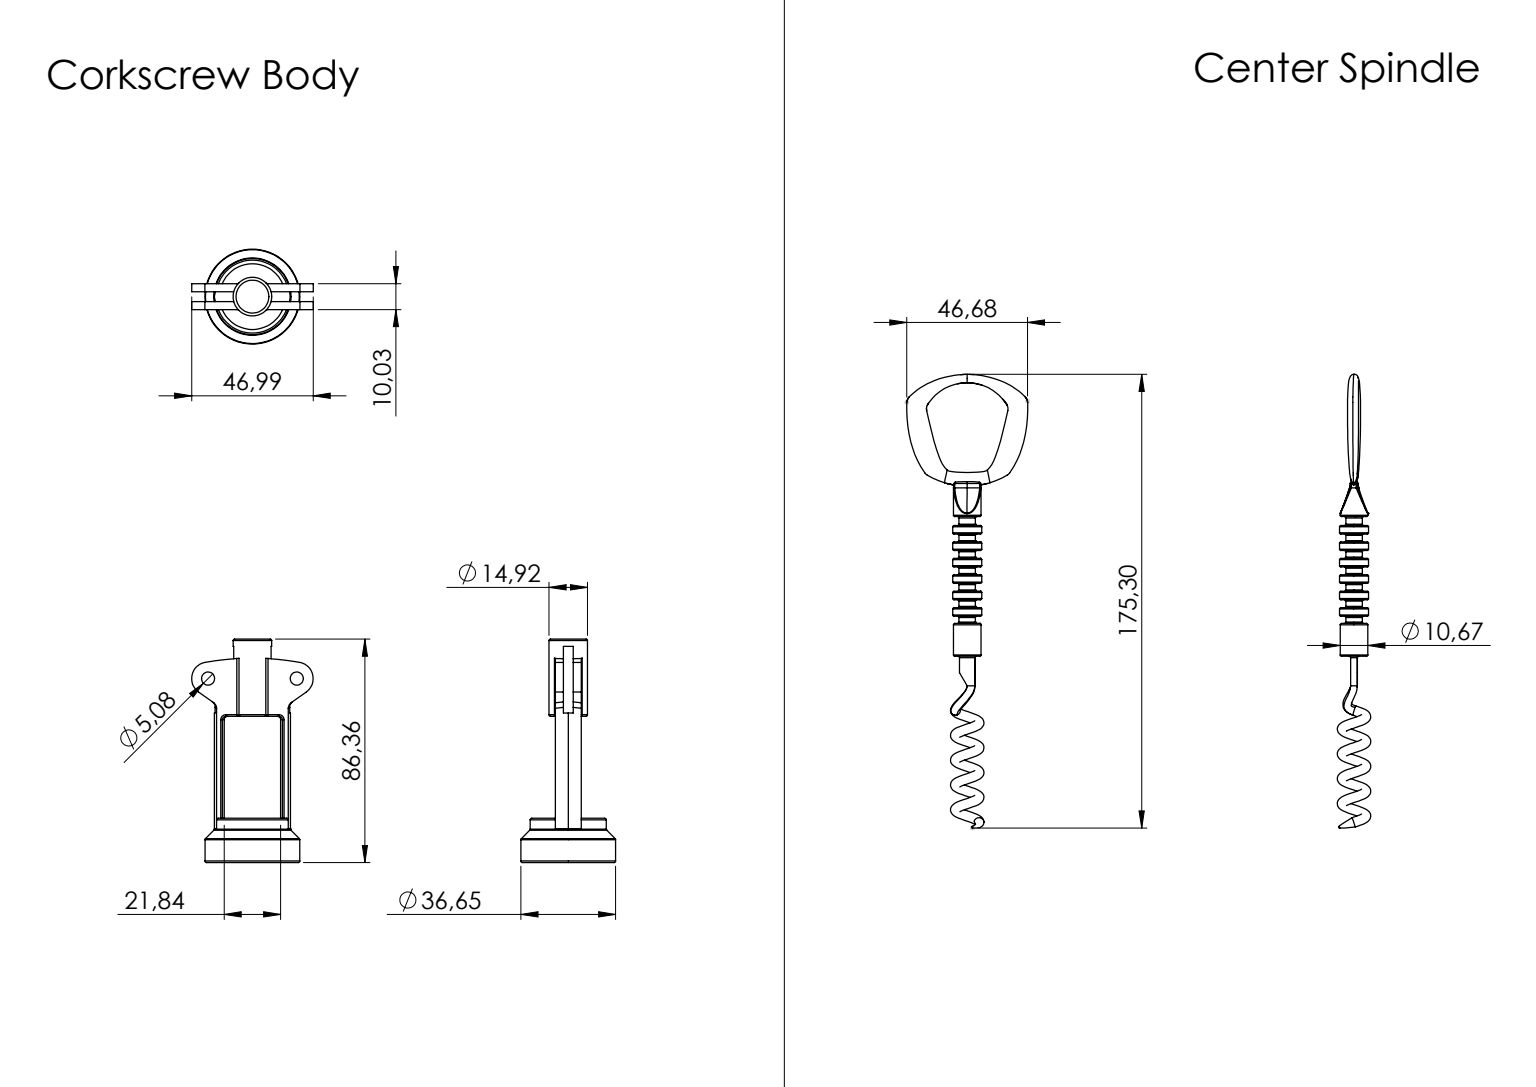
ISO-10303-21;
HEADER;
FILE_DESCRIPTION (('STEP AP214'),
    '1' );
FILE_NAME ('Corkscrew Body.step',
    '2026-10-06T14:27:08',
    ( '' ),
    ( '' ),
    'SwSTEP 2.0',
    'SolidWorks 2020',
    '' );
FILE_SCHEMA (( 'AUTOMOTIVE_DESIGN' ));
ENDSEC;

DATA;
#17=CARTESIAN_POINT ( 'NONE',  ( 16.60960244842765832, 9.026346327358513832, 0.000000000000000000 ) ) ;
#23=ORIENTED_EDGE ( 'NONE', *, *, #33925, .T. ) ;
#24=CIRCLE ( 'NONE', #38114, 2.540000000000000480 ) ;
#38=CYLINDRICAL_SURFACE ( 'NONE', #12263, 2.540000000000000480 ) ;
#46=CARTESIAN_POINT ( 'NONE',  ( -10.32169608105474090, 17.14500000000000313, 4.040823496909975887 ) ) ;
#53=DIRECTION ( 'NONE',  ( -1.000000000000000000, -9.933992704233682996E-16, 0.000000000000000000 ) ) ;
#54=CARTESIAN_POINT ( 'NONE',  ( 5.348924234570989533, 56.51499999999999346, 4.492130288940735738 ) ) ;
#63=CARTESIAN_POINT ( 'NONE',  ( 5.241362157049035631, 88.73331249999999670, 5.310945289804168468 ) ) ;
#81=AXIS2_PLACEMENT_3D ( 'NONE', #23637, #14261, #11485 ) ;
#83=CARTESIAN_POINT ( 'NONE',  ( -6.072850655491211391, 78.87349744216251679, 4.348040511725084656 ) ) ;
#86=EDGE_CURVE ( 'NONE', #35923, #21980, #18976, .T. ) ;
#92=CARTESIAN_POINT ( 'NONE',  ( 5.106395947886037234, 78.95054594174946772, -1.904999999999999583 ) ) ;
#107=VECTOR ( 'NONE', #35757, 1000.000000000000000 ) ;
#112=CARTESIAN_POINT ( 'NONE',  ( -5.241362157049125337, 53.58606250000000415, 5.310945289804168468 ) ) ;
#117=VERTEX_POINT ( 'NONE', #21192 ) ;
#125=CARTESIAN_POINT ( 'NONE',  ( 5.974493989214552769, 78.88147413144905329, -5.016499999999998849 ) ) ;
#143=CIRCLE ( 'NONE', #8295, 14.91798719394653716 ) ;
#166=ORIENTED_EDGE ( 'NONE', *, *, #11201, .F. ) ;
#183=FACE_OUTER_BOUND ( 'NONE', #18213, .T. ) ;
#195=DIRECTION ( 'NONE',  ( -1.000000000000000000, 9.627370216492861475E-17, 0.000000000000000000 ) ) ;
#199=CARTESIAN_POINT ( 'NONE',  ( -5.354045385512117505, 57.14999999999997726, -5.213862164334880589 ) ) ;
#207=PLANE ( 'NONE',  #933 ) ;
#222=CARTESIAN_POINT ( 'NONE',  ( -13.51785991797445341, 17.08228783296376818, -5.016500000000000625 ) ) ;
#244=CARTESIAN_POINT ( 'NONE',  ( -11.66725022231030628, 17.14499999999999957, -5.016499999999999737 ) ) ;
#248=ORIENTED_EDGE ( 'NONE', *, *, #30050, .T. ) ;
#268=CARTESIAN_POINT ( 'NONE',  ( -9.638062024671791406, 56.51499999999998636, 3.341163682266966022E-16 ) ) ;
#296=VERTEX_POINT ( 'NONE', #28017 ) ;
#299=ORIENTED_EDGE ( 'NONE', *, *, #22158, .F. ) ;
#305=CARTESIAN_POINT ( 'NONE',  ( -16.04309792416813707, 12.96416000000000146, 5.016499999999999737 ) ) ;
#306=ADVANCED_FACE ( 'NONE', ( #31428 ), #28233, .F. ) ;
#322=CARTESIAN_POINT ( 'NONE',  ( -5.305748947172281405, 65.30181249999996851, 5.247078976224250013 ) ) ;
#323=CARTESIAN_POINT ( 'NONE',  ( -14.73200000000000109, 57.78499999999998948, 0.000000000000000000 ) ) ;
#327=EDGE_CURVE ( 'NONE', #29906, #24559, #18939, .T. ) ;
#329=VERTEX_POINT ( 'NONE', #35268 ) ;
#344=DIRECTION ( 'NONE',  ( -1.000000000000000000, -6.353134868986659519E-16, 0.000000000000000000 ) ) ;
#359=VERTEX_POINT ( 'NONE', #29070 ) ;
#363=EDGE_CURVE ( 'NONE', #1559, #17444, #28654, .T. ) ;
#373=FACE_OUTER_BOUND ( 'NONE', #39695, .T. ) ;
#375=EDGE_CURVE ( 'NONE', #4024, #2187, #33931, .T. ) ;
#377=MECHANICAL_DESIGN_GEOMETRIC_PRESENTATION_REPRESENTATION('',(#2412),#24155);
#392=EDGE_CURVE ( 'NONE', #39604, #25560, #6092, .T. ) ;
#401=LINE ( 'NONE', #26358, #32745 ) ;
#406=EDGE_CURVE ( 'NONE', #11585, #11444, #23712, .T. ) ;
#415=CARTESIAN_POINT ( 'NONE',  ( -5.813542725971299063, 56.51499999999999346, -4.384680539058477322 ) ) ;
#431=CARTESIAN_POINT ( 'NONE',  ( -6.059261036834475256, 57.15000000000000568, 5.016499999999999737 ) ) ;
#433=EDGE_CURVE ( 'NONE', #15317, #27003, #40662, .T. ) ;
#449=VERTEX_POINT ( 'NONE', #15861 ) ;
#464=DIRECTION ( 'NONE',  ( 0.000000000000000000, 0.000000000000000000, 1.000000000000000000 ) ) ;
#479=CARTESIAN_POINT ( 'NONE',  ( -5.749535644243536581, 78.89971493812807068, 5.036102041843079746 ) ) ;
#482=CIRCLE ( 'NONE', #24259, 6.350000000000004974 ) ;
#493=ORIENTED_EDGE ( 'NONE', *, *, #10911, .T. ) ;
#506=CARTESIAN_POINT ( 'NONE',  ( -7.213960532363663525, 83.56599999999998829, -1.904999999999999805 ) ) ;
#532=CARTESIAN_POINT ( 'NONE',  ( -5.177913976931302287, 77.01756250000002524, 5.372099999999996989 ) ) ;
#552=CARTESIAN_POINT ( 'NONE',  ( 6.059261036834406866, 57.14999999999999858, -5.016499999999999737 ) ) ;
#583=CARTESIAN_POINT ( 'NONE',  ( 5.965356522962858676, 57.14999999999998437, 5.016499999999999737 ) ) ;
#584=ORIENTED_EDGE ( 'NONE', *, *, #327, .T. ) ;
#585=FACE_BOUND ( 'NONE', #36365, .T. ) ;
#586=EDGE_CURVE ( 'NONE', #26988, #6334, #37150, .T. ) ;
#605=CARTESIAN_POINT ( 'NONE',  ( 6.059261036834405978, 57.14999999999999858, 5.016500000000000625 ) ) ;
#609=CARTESIAN_POINT ( 'NONE',  ( -5.177913976931298734, 78.94499979771843812, 5.372100000000002318 ) ) ;
#619=ORIENTED_EDGE ( 'NONE', *, *, #5064, .T. ) ;
#627=CARTESIAN_POINT ( 'NONE',  ( -6.059261036834475256, 57.14999999999997016, -5.016499999999997961 ) ) ;
#644=EDGE_CURVE ( 'NONE', #33497, #18509, #30539, .T. ) ;
#660=ORIENTED_EDGE ( 'NONE', *, *, #1717, .T. ) ;
#672=ORIENTED_EDGE ( 'NONE', *, *, #20953, .T. ) ;
#676=DIRECTION ( 'NONE',  ( 6.353134868986659519E-16, -1.000000000000000000, -0.000000000000000000 ) ) ;
#677=EDGE_CURVE ( 'NONE', #32690, #22720, #25591, .T. ) ;
#681=CARTESIAN_POINT ( 'NONE',  ( 11.42297701379736097, 55.88459609804032624, 4.463034230327253660 ) ) ;
#688=CARTESIAN_POINT ( 'NONE',  ( -6.057513928997661168, 86.35999999999998522, 1.904999999999996030 ) ) ;
#700=VERTEX_POINT ( 'NONE', #35196 ) ;
#737=VECTOR ( 'NONE', #34279, 1000.000000000000000 ) ;
#738=EDGE_CURVE ( 'NONE', #20977, #19747, #15581, .T. ) ;
#739=CARTESIAN_POINT ( 'NONE',  ( -5.706177858098648414, 57.14999999999999147, 5.041924732081957572 ) ) ;
#740=CARTESIAN_POINT ( 'NONE',  ( -14.50851225146815615, 78.09971119798315442, -5.392902600000144986 ) ) ;
#747=ORIENTED_EDGE ( 'NONE', *, *, #36377, .F. ) ;
#772=ORIENTED_EDGE ( 'NONE', *, *, #41947, .T. ) ;
#798=CARTESIAN_POINT ( 'NONE',  ( 10.92199999999999704, 56.51500000000000057, 5.016499999999999737 ) ) ;
#815=EDGE_LOOP ( 'NONE', ( #35010, #24388, #10696, #2697 ) ) ;
#829=CARTESIAN_POINT ( 'NONE',  ( -18.10310074716289819, 60.88085900918027704, 4.514343177587270439 ) ) ;
#830=EDGE_CURVE ( 'NONE', #3380, #4530, #15208, .T. ) ;
#841=ORIENTED_EDGE ( 'NONE', *, *, #41067, .T. ) ;
#859=CARTESIAN_POINT ( 'NONE',  ( 5.965356522962838248, 88.73331249999999670, -5.016499999999999737 ) ) ;
#877=EDGE_CURVE ( 'NONE', #14016, #35273, #12805, .T. ) ;
#879=VECTOR ( 'NONE', #18768, 1000.000000000000000 ) ;
#883=CARTESIAN_POINT ( 'NONE',  ( 5.177913976931214357, 57.15000000000004832, 5.372099999999999653 ) ) ;
#884=ADVANCED_FACE ( 'NONE', ( #39437, #36878 ), #33047, .F. ) ;
#896=CARTESIAN_POINT ( 'NONE',  ( -5.285751105923923276, 78.93631598568865115, 5.267410652559463280 ) ) ;
#899=AXIS2_PLACEMENT_3D ( 'NONE', #27632, #8047, #4662 ) ;
#906=AXIS2_PLACEMENT_3D ( 'NONE', #17827, #7426, #24216 ) ;
#914=EDGE_CURVE ( 'NONE', #2471, #24940, #10804, .T. ) ;
#920=ADVANCED_FACE ( 'NONE', ( #1310 ), #35822, .T. ) ;
#922=AXIS2_PLACEMENT_3D ( 'NONE', #6804, #22543, #10198 ) ;
#926=VERTEX_POINT ( 'NONE', #17468 ) ;
#931=EDGE_CURVE ( 'NONE', #32109, #25746, #26433, .T. ) ;
#932=CARTESIAN_POINT ( 'NONE',  ( 11.11710224467026542, 56.30409367656755393, -5.016499999999892268 ) ) ;
#933=AXIS2_PLACEMENT_3D ( 'NONE', #16577, #26595, #39603 ) ;
#934=ADVANCED_FACE ( 'NONE', ( #10661 ), #17435, .T. ) ;
#950=CARTESIAN_POINT ( 'NONE',  ( -4.965996940879724875, 56.51500000000000767, 4.710730864944216556 ) ) ;
#970=DIRECTION ( 'NONE',  ( -0.8138664877804109299, 0.5810519254489895369, 0.000000000000000000 ) ) ;
#1007=VERTEX_POINT ( 'NONE', #36453 ) ;
#1017=CARTESIAN_POINT ( 'NONE',  ( 6.059261036833978764, 78.87450423423040036, 5.016499999999999737 ) ) ;
#1029=ORIENTED_EDGE ( 'NONE', *, *, #32030, .T. ) ;
#1042=COLOUR_RGB ( '', 0.08235294, 0.09019608, 0.10196078) ;
#1052=ORIENTED_EDGE ( 'NONE', *, *, #4297, .T. ) ;
#1067=CARTESIAN_POINT ( 'NONE',  ( 5.475330206976798841, 65.30181249999998272, -5.107412922131463695 ) ) ;
#1086=EDGE_CURVE ( 'NONE', #24253, #32761, #16627, .T. ) ;
#1089=CYLINDRICAL_SURFACE ( 'NONE', #27471, 14.73199999999999577 ) ;
#1109=CARTESIAN_POINT ( 'NONE',  ( -5.153324091253895567, 56.51694919289731445, -4.640537933314518249 ) ) ;
#1121=EDGE_LOOP ( 'NONE', ( #34298, #24074 ) ) ;
#1132=ADVANCED_FACE ( 'NONE', ( #40076 ), #32397, .T. ) ;
#1152=FACE_OUTER_BOUND ( 'NONE', #15557, .T. ) ;
#1157=LINE ( 'NONE', #36934, #4914 ) ;
#1161=VECTOR ( 'NONE', #11393, 1000.000000000000000 ) ;
#1166=ORIENTED_EDGE ( 'NONE', *, *, #32177, .F. ) ;
#1177=CARTESIAN_POINT ( 'NONE',  ( -14.73199999999999754, 61.59499999999999886, 5.016499999999999737 ) ) ;
#1205=EDGE_CURVE ( 'NONE', #21382, #34762, #21073, .T. ) ;
#1209=CARTESIAN_POINT ( 'NONE',  ( -11.66725022231030984, 16.50999999999999801, 5.016499999999999737 ) ) ;
#1242=ORIENTED_EDGE ( 'NONE', *, *, #38846, .T. ) ;
#1250=CARTESIAN_POINT ( 'NONE',  ( 14.60500000000000043, 71.11999999999999034, -1.904999999999999583 ) ) ;
#1264=FACE_OUTER_BOUND ( 'NONE', #33978, .T. ) ;
#1296=DIRECTION ( 'NONE',  ( 9.627370216492862708E-17, 1.000000000000000000, -0.000000000000000000 ) ) ;
#1307=CYLINDRICAL_SURFACE ( 'NONE', #5741, 18.32410244842765934 ) ;
#1308=VECTOR ( 'NONE', #32914, 1000.000000000000000 ) ;
#1310=FACE_OUTER_BOUND ( 'NONE', #18095, .T. ) ;
#1313=ORIENTED_EDGE ( 'NONE', *, *, #40737, .T. ) ;
#1327=ORIENTED_EDGE ( 'NONE', *, *, #33725, .F. ) ;
#1357=AXIS2_PLACEMENT_3D ( 'NONE', #16330, #30595, #17389 ) ;
#1371=ORIENTED_EDGE ( 'NONE', *, *, #327, .F. ) ;
#1374=VERTEX_POINT ( 'NONE', #11919 ) ;
#1386=ORIENTED_EDGE ( 'NONE', *, *, #433, .F. ) ;
#1397=VERTEX_POINT ( 'NONE', #25016 ) ;
#1404=DIRECTION ( 'NONE',  ( -0.000000000000000000, -0.000000000000000000, -1.000000000000000000 ) ) ;
#1422=VERTEX_POINT ( 'NONE', #19455 ) ;
#1427=PLANE ( 'NONE',  #33605 ) ;
#1454=FACE_OUTER_BOUND ( 'NONE', #20510, .T. ) ;
#1460=DIRECTION ( 'NONE',  ( -1.000000000000000000, 0.000000000000000000, 0.000000000000000000 ) ) ;
#1463=EDGE_CURVE ( 'NONE', #18019, #32240, #9670, .T. ) ;
#1466=AXIS2_PLACEMENT_3D ( 'NONE', #18039, #21025, #19252 ) ;
#1485=DIRECTION ( 'NONE',  ( 9.627370216492862708E-17, 1.000000000000000000, -0.000000000000000000 ) ) ;
#1489=CARTESIAN_POINT ( 'NONE',  ( 5.965356522962860453, 65.30181249999998272, -5.016499999999999737 ) ) ;
#1511=ORIENTED_EDGE ( 'NONE', *, *, #11811, .F. ) ;
#1514=CARTESIAN_POINT ( 'NONE',  ( 12.21488373879589240, 17.14499999999999957, 4.381499999999999950 ) ) ;
#1519=CARTESIAN_POINT ( 'NONE',  ( 9.925711944554073796, 78.55658865046544292, -5.016499999999999737 ) ) ;
#1529=CARTESIAN_POINT ( 'NONE',  ( -11.37822013471355653, 56.06794068206369275, -5.016499999999995296 ) ) ;
#1531=CIRCLE ( 'NONE', #25317, 18.13811525448111439 ) ;
#1533=CARTESIAN_POINT ( 'NONE',  ( 1.247998466936322838E-15, 12.96302561210691806, 0.000000000000000000 ) ) ;
#1544=VERTEX_POINT ( 'NONE', #29261 ) ;
#1559=VERTEX_POINT ( 'NONE', #16682 ) ;
#1561=CARTESIAN_POINT ( 'NONE',  ( 10.45722248778832508, 56.52709681235301531, -5.016500000000866599 ) ) ;
#1573=VECTOR ( 'NONE', #21848, 999.9999999999998863 ) ;
#1616=DIRECTION ( 'NONE',  ( -1.000000000000000000, -6.353134868986659519E-16, 6.146657985744592735E-16 ) ) ;
#1628=ORIENTED_EDGE ( 'NONE', *, *, #19844, .T. ) ;
#1638=LINE ( 'NONE', #34216, #5021 ) ;
#1675=AXIS2_PLACEMENT_3D ( 'NONE', #6302, #35478, #19903 ) ;
#1699=DIRECTION ( 'NONE',  ( 0.1469470846586743706, 0.000000000000000000, 0.9891443546370348727 ) ) ;
#1717=EDGE_CURVE ( 'NONE', #31005, #40327, #26908, .T. ) ;
#1727=ADVANCED_FACE ( 'NONE', ( #1152 ), #40132, .T. ) ;
#1735=DIRECTION ( 'NONE',  ( -1.000000000000000000, 0.000000000000000000, -6.146657985744586818E-16 ) ) ;
#1749=EDGE_CURVE ( 'NONE', #19747, #35348, #13067, .T. ) ;
#1755=FILL_AREA_STYLE_COLOUR ( '', #18907 ) ;
#1769=AXIS2_PLACEMENT_3D ( 'NONE', #10155, #36381, #23767 ) ;
#1787=CARTESIAN_POINT ( 'NONE',  ( 4.792324638223571576, 56.51998046905274009, -4.972049999999996750 ) ) ;
#1816=LINE ( 'NONE', #30764, #8889 ) ;
#1830=ORIENTED_EDGE ( 'NONE', *, *, #17540, .F. ) ;
#1833=DIRECTION ( 'NONE',  ( -0.000000000000000000, -0.000000000000000000, -1.000000000000000000 ) ) ;
#1848=DIRECTION ( 'NONE',  ( -1.000000000000000000, -5.463695987328526437E-16, 0.000000000000000000 ) ) ;
#1874=DIRECTION ( 'NONE',  ( -0.000000000000000000, -0.000000000000000000, -1.000000000000000000 ) ) ;
#1876=CARTESIAN_POINT ( 'NONE',  ( 6.059261036834405978, 56.51500000000000057, -5.016500000000000625 ) ) ;
#1883=VERTEX_POINT ( 'NONE', #18570 ) ;
#1892=ORIENTED_EDGE ( 'NONE', *, *, #31827, .F. ) ;
#1907=VECTOR ( 'NONE', #2855, 1000.000000000000000 ) ;
#1910=ADVANCED_FACE ( 'NONE', ( #37755 ), #18355, .F. ) ;
#1923=DIRECTION ( 'NONE',  ( -1.000000000000000000, 0.000000000000000000, 0.000000000000000000 ) ) ;
#1930=CARTESIAN_POINT ( 'NONE',  ( -5.177913976931281859, 56.51500000000002899, -5.372099999999998765 ) ) ;
#1935=CYLINDRICAL_SURFACE ( 'NONE', #12373, 2.539999999999999591 ) ;
#1942=CARTESIAN_POINT ( 'NONE',  ( -11.66725022231030628, 55.24499999999998323, -5.016500000000000625 ) ) ;
#1962=SURFACE_SIDE_STYLE ('',( #8555 ) ) ;
#1964=DIRECTION ( 'NONE',  ( 1.000000000000000000, 0.000000000000000000, 1.224646799147353207E-16 ) ) ;
#1968=DIRECTION ( 'NONE',  ( -6.353134868986659519E-16, 1.000000000000000000, 0.000000000000000000 ) ) ;
#1976=FACE_OUTER_BOUND ( 'NONE', #17302, .T. ) ;
#2000=CIRCLE ( 'NONE', #24436, 12.69999999999999751 ) ;
#2012=DIRECTION ( 'NONE',  ( 0.9849462604886048966, -0.000000000000000000, 0.1728608224830406881 ) ) ;
#2044=ORIENTED_EDGE ( 'NONE', *, *, #9457, .T. ) ;
#2049=CARTESIAN_POINT ( 'NONE',  ( 5.230039278750658660, 78.94094791484917550, -5.321858878493932465 ) ) ;
#2057=CARTESIAN_POINT ( 'NONE',  ( -5.817775060672866871, 56.51499999999999346, -4.384522920466269014 ) ) ;
#2074=ORIENTED_EDGE ( 'NONE', *, *, #375, .F. ) ;
#2078=FACE_OUTER_BOUND ( 'NONE', #34790, .T. ) ;
#2083=EDGE_CURVE ( 'NONE', #14687, #5970, #12181, .T. ) ;
#2085=CARTESIAN_POINT ( 'NONE',  ( 5.115576404397946142, 56.51499999999996504, -4.603576161448420301 ) ) ;
#2088=VECTOR ( 'NONE', #7580, 1000.000000000000227 ) ;
#2098=DIRECTION ( 'NONE',  ( -1.000000000000000000, 0.000000000000000000, 0.000000000000000000 ) ) ;
#2108=DIRECTION ( 'NONE',  ( 0.8138664877804110409, 0.5810519254489896479, -5.002558946445370251E-16 ) ) ;
#2110=LINE ( 'NONE', #34903, #737 ) ;
#2132=FACE_OUTER_BOUND ( 'NONE', #16740, .T. ) ;
#2134=EDGE_CURVE ( 'NONE', #25560, #18746, #14952, .T. ) ;
#2138=CIRCLE ( 'NONE', #30043, 12.69999999999999751 ) ;
#2141=CARTESIAN_POINT ( 'NONE',  ( -14.73199999999999399, 12.96302561210691984, 0.000000000000000000 ) ) ;
#2145=ORIENTED_EDGE ( 'NONE', *, *, #40646, .F. ) ;
#2146=DIRECTION ( 'NONE',  ( -1.000000000000000000, 0.000000000000000000, 0.000000000000000000 ) ) ;
#2150=DIRECTION ( 'NONE',  ( 0.000000000000000000, 0.000000000000000000, -1.000000000000000000 ) ) ;
#2153=LINE ( 'NONE', #15113, #21689 ) ;
#2164=EDGE_LOOP ( 'NONE', ( #13314, #38087, #29660, #7685 ) ) ;
#2177=DIRECTION ( 'NONE',  ( -0.9849462604886047856, 0.000000000000000000, -0.1728608224830407714 ) ) ;
#2187=VERTEX_POINT ( 'NONE', #12611 ) ;
#2189=FACE_OUTER_BOUND ( 'NONE', #17505, .T. ) ;
#2204=DIRECTION ( 'NONE',  ( -1.000000000000000000, 0.000000000000000000, 0.000000000000000000 ) ) ;
#2209=CARTESIAN_POINT ( 'NONE',  ( 5.177913976931212581, 57.15000000000004832, -5.372100000000001430 ) ) ;
#2215=AXIS2_PLACEMENT_3D ( 'NONE', #11347, #15162, #11767 ) ;
#2216=ORIENTED_EDGE ( 'NONE', *, *, #20706, .T. ) ;
#2248=CARTESIAN_POINT ( 'NONE',  ( -6.985000000000036735, 57.14999999999998437, 0.000000000000000000 ) ) ;
#2252=LINE ( 'NONE', #11602, #31088 ) ;
#2260=FACE_OUTER_BOUND ( 'NONE', #37704, .T. ) ;
#2266=DIRECTION ( 'NONE',  ( 1.000000000000000000, -1.162840169671635117E-16, 0.000000000000000000 ) ) ;
#2274=CARTESIAN_POINT ( 'NONE',  ( 5.177913976931196594, 78.94499979771845233, -5.372100000000001430 ) ) ;
#2296=VECTOR ( 'NONE', #9251, 1000.000000000000000 ) ;
#2302=CARTESIAN_POINT ( 'NONE',  ( 5.860205464978446521, 56.51500000000089585, -5.019550312247728741 ) ) ;
#2314=CARTESIAN_POINT ( 'NONE',  ( -17.68910244842765778, 8.844871939465427602, 2.166290269325653984E-15 ) ) ;
#2341=VECTOR ( 'NONE', #1296, 1000.000000000000000 ) ;
#2349=AXIS2_PLACEMENT_3D ( 'NONE', #22246, #26089, #344 ) ;
#2350=PLANE ( 'NONE',  #8239 ) ;
#2354=CARTESIAN_POINT ( 'NONE',  ( -12.16475753114683656, 55.74362973025081658, 5.016499999999999737 ) ) ;
#2357=DIRECTION ( 'NONE',  ( -1.000000000000000000, -9.933992704233682996E-16, 0.000000000000000000 ) ) ;
#2359=ORIENTED_EDGE ( 'NONE', *, *, #37833, .F. ) ;
#2369=DIRECTION ( 'NONE',  ( -1.224646799147353207E-16, 1.179012811983454535E-32, 1.000000000000000000 ) ) ;
#2378=ORIENTED_EDGE ( 'NONE', *, *, #677, .T. ) ;
#2384=EDGE_CURVE ( 'NONE', #36071, #117, #19612, .T. ) ;
#2391=DIRECTION ( 'NONE',  ( 6.353134868986659519E-16, -1.000000000000000000, 0.000000000000000000 ) ) ;
#2411=EDGE_CURVE ( 'NONE', #7919, #11738, #39022, .T. ) ;
#2412=STYLED_ITEM ( 'NONE', ( #26181 ), #38952 ) ;
#2421=CARTESIAN_POINT ( 'NONE',  ( 10.92199999999999704, 16.51000000000000156, 5.016499999999999737 ) ) ;
#2425=ORIENTED_EDGE ( 'NONE', *, *, #35443, .F. ) ;
#2440=B_SPLINE_SURFACE_WITH_KNOTS ( 'NONE', 3, 1, ( 
 ( #6364, #2966 ),
 ( #22726, #38531 ),
 ( #26158, #13168 ),
 ( #15929, #28725 ) ),
 .UNSPECIFIED., .F., .F., .F.,
 ( 4, 4 ),
 ( 2, 2 ),
 ( 0.000000000000000000, 0.6118630412642164229 ),
 ( 0.000000000000000000, 1.000000000000000000 ),
 .UNSPECIFIED. ) ;
#2448=ORIENTED_EDGE ( 'NONE', *, *, #21122, .T. ) ;
#2466=EDGE_CURVE ( 'NONE', #35912, #359, #33547, .T. ) ;
#2467=CARTESIAN_POINT ( 'NONE',  ( -5.965356522962950159, 77.01756249999996840, -5.016499999999999737 ) ) ;
#2470=VECTOR ( 'NONE', #25773, 999.9999999999998863 ) ;
#2471=VERTEX_POINT ( 'NONE', #33268 ) ;
#2474=DIRECTION ( 'NONE',  ( -1.000000000000000000, 9.627370216492862708E-17, 0.000000000000000000 ) ) ;
#2480=DIRECTION ( 'NONE',  ( 0.000000000000000000, 0.000000000000000000, -1.000000000000000000 ) ) ;
#2487=PLANE ( 'NONE',  #4772 ) ;
#2488=EDGE_CURVE ( 'NONE', #18952, #41795, #38005, .T. ) ;
#2517=CARTESIAN_POINT ( 'NONE',  ( 5.652760403059779115, 78.90762248850970195, 4.881857480398483773 ) ) ;
#2518=EDGE_CURVE ( 'NONE', #38485, #22696, #17475, .T. ) ;
#2521=EDGE_CURVE ( 'NONE', #19034, #29525, #10668, .T. ) ;
#2547=ORIENTED_EDGE ( 'NONE', *, *, #22871, .F. ) ;
#2554=VECTOR ( 'NONE', #26088, 1000.000000000000000 ) ;
#2559=CARTESIAN_POINT ( 'NONE',  ( 1.650612623617701454E-15, 17.14499999999999957, 0.000000000000000000 ) ) ;
#2560=AXIS2_PLACEMENT_3D ( 'NONE', #26322, #10762, #36974 ) ;
#2561=DIRECTION ( 'NONE',  ( 0.000000000000000000, -0.000000000000000000, -1.000000000000000000 ) ) ;
#2567=CARTESIAN_POINT ( 'NONE',  ( 5.237865101059586692, 78.94033958618257429, 5.314315937239232568 ) ) ;
#2583=DIRECTION ( 'NONE',  ( -0.000000000000000000, -0.000000000000000000, -1.000000000000000000 ) ) ;
#2628=CARTESIAN_POINT ( 'NONE',  ( -5.266289895157169814E-14, 83.56599999999998829, 1.904999999999999805 ) ) ;
#2631=PLANE ( 'NONE',  #39625 ) ;
#2695=CARTESIAN_POINT ( 'NONE',  ( 12.21488373879589240, 71.11999999999999034, 5.016499999999999737 ) ) ;
#2696=CARTESIAN_POINT ( 'NONE',  ( 5.177913976931201923, 71.67999986514567468, -5.372100000000002318 ) ) ;
#2697=ORIENTED_EDGE ( 'NONE', *, *, #29178, .F. ) ;
#2707=EDGE_CURVE ( 'NONE', #32109, #11189, #16941, .T. ) ;
#2711=AXIS2_PLACEMENT_3D ( 'NONE', #25509, #5513, #21659 ) ;
#2719=DIRECTION ( 'NONE',  ( -0.000000000000000000, -0.000000000000000000, -1.000000000000000000 ) ) ;
#2724=CARTESIAN_POINT ( 'NONE',  ( 5.353961913965608055, 57.14999999999869829, -5.213928161019547147 ) ) ;
#2728=FACE_OUTER_BOUND ( 'NONE', #31465, .T. ) ;
#2731=CIRCLE ( 'NONE', #26532, 12.69999999999999751 ) ;
#2754=ORIENTED_EDGE ( 'NONE', *, *, #4976, .F. ) ;
#2757=EDGE_CURVE ( 'NONE', #3380, #22739, #11186, .T. ) ;
#2767=ADVANCED_FACE ( 'NONE', ( #33780 ), #30564, .F. ) ;
#2771=CARTESIAN_POINT ( 'NONE',  ( -11.58677707360117282, 55.41127257906216386, 4.474811398756911807 ) ) ;
#2772=CARTESIAN_POINT ( 'NONE',  ( 5.624629865489175096, 78.90958242041968163, 5.067363953418781541 ) ) ;
#2776=CARTESIAN_POINT ( 'NONE',  ( 18.10310074716289819, 60.88085900918027704, 4.514343177587270439 ) ) ;
#2779=ORIENTED_EDGE ( 'NONE', *, *, #9655, .T. ) ;
#2792=FILL_AREA_STYLE_COLOUR ( '', #1042 ) ;
#2794=CARTESIAN_POINT ( 'NONE',  ( -6.985000000000036735, 56.51499999999998636, 0.000000000000000000 ) ) ;
#2803=ORIENTED_EDGE ( 'NONE', *, *, #2521, .F. ) ;
#2804=EDGE_LOOP ( 'NONE', ( #15092, #6381, #25239, #7806 ) ) ;
#2819=AXIS2_PLACEMENT_3D ( 'NONE', #38175, #21956, #5807 ) ;
#2827=CARTESIAN_POINT ( 'NONE',  ( -5.177913976931298734, 78.94499979771843812, -5.372100000000003206 ) ) ;
#2834=CARTESIAN_POINT ( 'NONE',  ( -10.39017547737320157, 56.51499999999998636, 6.098637220230963427E-16 ) ) ;
#2838=DIRECTION ( 'NONE',  ( 1.000000000000000000, 0.000000000000000000, 0.000000000000000000 ) ) ;
#2852=ORIENTED_EDGE ( 'NONE', *, *, #6404, .T. ) ;
#2855=DIRECTION ( 'NONE',  ( 0.000000000000000000, 1.000000000000000000, 0.000000000000000000 ) ) ;
#2857=CARTESIAN_POINT ( 'NONE',  ( 17.14499999999999957, 71.11999999999999034, 5.016499999999999737 ) ) ;
#2862=ORIENTED_EDGE ( 'NONE', *, *, #3971, .T. ) ;
#2869=CARTESIAN_POINT ( 'NONE',  ( 14.50851225146812240, 78.09971119798316863, -1.904999999999999583 ) ) ;
#2872=DIRECTION ( 'NONE',  ( 6.353134868986659519E-16, -1.000000000000000000, 0.000000000000000000 ) ) ;
#2882=CARTESIAN_POINT ( 'NONE',  ( -5.475330206976867231, 65.30181249999998272, -5.107412922131463695 ) ) ;
#2888=EDGE_CURVE ( 'NONE', #8736, #12419, #14571, .T. ) ;
#2895=DIRECTION ( 'NONE',  ( -9.627370216492862708E-17, -1.000000000000000000, 0.000000000000000000 ) ) ;
#2899=CARTESIAN_POINT ( 'NONE',  ( 10.86251533436410277, 78.45482716897161879, 1.904999999999999583 ) ) ;
#2905=EDGE_LOOP ( 'NONE', ( #38246, #11736, #28782, #1830 ) ) ;
#2912=EDGE_CURVE ( 'NONE', #2187, #21980, #1816, .T. ) ;
#2918=CARTESIAN_POINT ( 'NONE',  ( -10.92199999999999704, 12.96416000000000146, 0.000000000000000000 ) ) ;
#2920=ORIENTED_EDGE ( 'NONE', *, *, #2488, .F. ) ;
#2934=ORIENTED_EDGE ( 'NONE', *, *, #1749, .T. ) ;
#2952=AXIS2_PLACEMENT_3D ( 'NONE', #5972, #19351, #38343 ) ;
#2966=CARTESIAN_POINT ( 'NONE',  ( 18.35410564743290962, 77.35382415001784295, 1.904999999999988258 ) ) ;
#2972=CARTESIAN_POINT ( 'NONE',  ( -5.449227423685445437, 56.51500000000039847, -5.145694933558188744 ) ) ;
#2975=CARTESIAN_POINT ( 'NONE',  ( 5.654802103384407808, 78.90710107780496685, 5.057831774704117045 ) ) ;
#2997=CARTESIAN_POINT ( 'NONE',  ( -9.665786669610962889, 55.24499999999999034, 0.1866227975165204167 ) ) ;
#3003=DIRECTION ( 'NONE',  ( -1.000000000000000000, 1.288607544181256696E-16, 0.000000000000000000 ) ) ;
#3029=EDGE_CURVE ( 'NONE', #14963, #32351, #15483, .T. ) ;
#3030=DIRECTION ( 'NONE',  ( -1.000000000000000000, 0.000000000000000000, 0.000000000000000000 ) ) ;
#3036=CARTESIAN_POINT ( 'NONE',  ( -11.58677707360137532, 17.14499999999999957, 4.474811398758258285 ) ) ;
#3052=ORIENTED_EDGE ( 'NONE', *, *, #1205, .T. ) ;
#3054=( BOUNDED_CURVE ( )  B_SPLINE_CURVE ( 3, ( #28704, #41713, #12519, #28909 ),
 .UNSPECIFIED., .F., .T. ) 
 B_SPLINE_CURVE_WITH_KNOTS ( ( 4, 4 ),
 ( 4.712388980384686121, 5.673871460451326065 ),
 .UNSPECIFIED. ) 
 CURVE ( )  GEOMETRIC_REPRESENTATION_ITEM ( )  RATIONAL_B_SPLINE_CURVE ( ( 1.000000000000000000, 0.9244349266169030743, 0.9244349266169030743, 1.000000000000000000 ) ) 
 REPRESENTATION_ITEM ( '' )  );
#3062=ORIENTED_EDGE ( 'NONE', *, *, #26982, .T. ) ;
#3074=ORIENTED_EDGE ( 'NONE', *, *, #3776, .T. ) ;
#3090=LINE ( 'NONE', #19457, #7963 ) ;
#3110=CARTESIAN_POINT ( 'NONE',  ( -10.92199999999999704, 55.24499999999999034, -7.690731210240437325E-16 ) ) ;
#3156=CARTESIAN_POINT ( 'NONE',  ( 4.825844303143274949, 56.51499999999997215, 4.829557277217847222 ) ) ;
#3161=ORIENTED_EDGE ( 'NONE', *, *, #5173, .T. ) ;
#3167=VERTEX_POINT ( 'NONE', #323 ) ;
#3169=DIRECTION ( 'NONE',  ( -1.000000000000000000, -6.353134868986659519E-16, 0.000000000000000000 ) ) ;
#3176=CARTESIAN_POINT ( 'NONE',  ( 5.594725610051233922, 78.91206791035247647, 5.077866005995121057 ) ) ;
#3183=FACE_BOUND ( 'NONE', #18284, .T. ) ;
#3184=AXIS2_PLACEMENT_3D ( 'NONE', #23963, #20974, #13964 ) ;
#3185=ORIENTED_EDGE ( 'NONE', *, *, #35246, .F. ) ;
#3193=CARTESIAN_POINT ( 'NONE',  ( -6.059261036834476144, 56.58343591620776181, 4.712961528314683513 ) ) ;
#3198=FACE_OUTER_BOUND ( 'NONE', #31075, .T. ) ;
#3225=ADVANCED_FACE ( 'NONE', ( #2728 ), #13858, .T. ) ;
#3228=ORIENTED_EDGE ( 'NONE', *, *, #6639, .F. ) ;
#3231=LINE ( 'NONE', #13229, #9569 ) ;
#3234=CARTESIAN_POINT ( 'NONE',  ( -16.04309792416813707, 12.96416000000000146, 5.016499999999999737 ) ) ;
#3239=DIRECTION ( 'NONE',  ( 0.1469470846586743706, -1.414713986243376972E-17, 0.9891443546370348727 ) ) ;
#3251=DIRECTION ( 'NONE',  ( 9.627370216492862708E-17, 1.000000000000000000, -0.000000000000000000 ) ) ;
#3255=CIRCLE ( 'NONE', #27716, 6.350000000000004974 ) ;
#3259=DIRECTION ( 'NONE',  ( 6.353134868986659519E-16, -1.000000000000000000, 0.000000000000000000 ) ) ;
#3269=DIRECTION ( 'NONE',  ( -1.000000000000000000, 1.044409991968846932E-16, 0.000000000000000000 ) ) ;
#3274=CARTESIAN_POINT ( 'NONE',  ( -5.653927021192587610, 78.90752773945908416, 4.880377097574616130 ) ) ;
#3275=AXIS2_PLACEMENT_3D ( 'NONE', #6670, #19223, #39468 ) ;
#3284=CARTESIAN_POINT ( 'NONE',  ( 14.50851225146812240, 78.09971119798316863, -5.392902600000141433 ) ) ;
#3292=ORIENTED_EDGE ( 'NONE', *, *, #3466, .T. ) ;
#3321=DIRECTION ( 'NONE',  ( -0.1469470846586743706, 1.414713986243376972E-17, -0.9891443546370348727 ) ) ;
#3326=AXIS2_PLACEMENT_3D ( 'NONE', #13453, #16635, #4514 ) ;
#3339=ORIENTED_EDGE ( 'NONE', *, *, #25682, .F. ) ;
#3363=LINE ( 'NONE', #6762, #28527 ) ;
#3365=AXIS2_PLACEMENT_3D ( 'NONE', #37717, #35158, #38560 ) ;
#3370=CARTESIAN_POINT ( 'NONE',  ( 5.449227423779250401, 57.14999999999996305, 5.145694933688582218 ) ) ;
#3377=DIRECTION ( 'NONE',  ( 1.000000000000000000, 1.004817652842027660E-15, 0.000000000000000000 ) ) ;
#3379=ADVANCED_FACE ( 'NONE', ( #14538 ), #7331, .F. ) ;
#3380=VERTEX_POINT ( 'NONE', #37341 ) ;
#3382=CARTESIAN_POINT ( 'NONE',  ( 6.113380087472956159E-17, 0.6350000000000001199, 0.000000000000000000 ) ) ;
#3388=CARTESIAN_POINT ( 'NONE',  ( -13.85159022459153988, 59.63164443796365077, 5.016499999999999737 ) ) ;
#3391=CARTESIAN_POINT ( 'NONE',  ( 5.736468567008338404, 78.90050738914777639, 5.037638016205330693 ) ) ;
#3392=CARTESIAN_POINT ( 'NONE',  ( 16.04309792416813707, 12.96416000000000146, 5.016499999999999737 ) ) ;
#3396=CARTESIAN_POINT ( 'NONE',  ( -5.654802103384504619, 78.90710107780492422, -5.057831774704119709 ) ) ;
#3409=CARTESIAN_POINT ( 'NONE',  ( -13.83234216238653858, 16.68269501491596785, -5.016499999999998849 ) ) ;
#3424=EDGE_CURVE ( 'NONE', #33118, #4862, #30711, .T. ) ;
#3426=ORIENTED_EDGE ( 'NONE', *, *, #30280, .F. ) ;
#3434=EDGE_CURVE ( 'NONE', #31942, #3896, #27315, .T. ) ;
#3445=CYLINDRICAL_SURFACE ( 'NONE', #40339, 2.539999999999999591 ) ;
#3466=EDGE_CURVE ( 'NONE', #16450, #8022, #18188, .T. ) ;
#3470=CARTESIAN_POINT ( 'NONE',  ( 5.965356522962860453, 53.58606249999999704, 5.016499999999999737 ) ) ;
#3477=EDGE_CURVE ( 'NONE', #20581, #20298, #10043, .T. ) ;
#3499=FACE_OUTER_BOUND ( 'NONE', #20995, .T. ) ;
#3509=ORIENTED_EDGE ( 'NONE', *, *, #4350, .T. ) ;
#3510=CARTESIAN_POINT ( 'NONE',  ( 7.017589760824501255, 78.79342665089201603, 2.556811674275345059 ) ) ;
#3515=CARTESIAN_POINT ( 'NONE',  ( -5.965356522962950159, 88.73331249999998249, 5.016499999999999737 ) ) ;
#3521=ORIENTED_EDGE ( 'NONE', *, *, #15903, .T. ) ;
#3538=CARTESIAN_POINT ( 'NONE',  ( 5.965356522962859565, 57.14999999999999858, -5.016499999999999737 ) ) ;
#3557=DIRECTION ( 'NONE',  ( 0.000000000000000000, -1.000000000000000000, 0.000000000000000000 ) ) ;
#3594=ORIENTED_EDGE ( 'NONE', *, *, #6327, .T. ) ;
#3599=ORIENTED_EDGE ( 'NONE', *, *, #37027, .T. ) ;
#3607=CARTESIAN_POINT ( 'NONE',  ( -14.95453923199683643, 61.75387968257833649, 5.016499999999999737 ) ) ;
#3614=CARTESIAN_POINT ( 'NONE',  ( -5.594725610051334286, 78.91206791035253332, -5.077866005995125498 ) ) ;
#3628=SURFACE_STYLE_USAGE ( .BOTH. , #6808 ) ;
#3634=CARTESIAN_POINT ( 'NONE',  ( 19.68500000000000227, 71.11999999999999034, -5.016499999999999737 ) ) ;
#3641=VERTEX_POINT ( 'NONE', #26017 ) ;
#3652=ORIENTED_EDGE ( 'NONE', *, *, #11204, .F. ) ;
#3656=CARTESIAN_POINT ( 'NONE',  ( -3.590790587123838709E-14, 56.51998046905274009, 0.000000000000000000 ) ) ;
#3657=AXIS2_PLACEMENT_3D ( 'NONE', #25269, #18657, #38482 ) ;
#3678=ADVANCED_FACE ( 'NONE', ( #6236 ), #19206, .F. ) ;
#3684=ORIENTED_EDGE ( 'NONE', *, *, #15651, .F. ) ;
#3698=DIRECTION ( 'NONE',  ( 6.353134868986659519E-16, -1.000000000000000000, 0.000000000000000000 ) ) ;
#3716=VECTOR ( 'NONE', #19059, 1000.000000000000000 ) ;
#3719=CARTESIAN_POINT ( 'NONE',  ( -10.28897677580358305, 57.14999999999998437, 5.016499999999999737 ) ) ;
#3733=ORIENTED_EDGE ( 'NONE', *, *, #22706, .T. ) ;
#3744=CARTESIAN_POINT ( 'NONE',  ( 11.58677707360137532, 17.14500000000046498, -4.474811398758258285 ) ) ;
#3749=CARTESIAN_POINT ( 'NONE',  ( 14.73199999999999754, 61.59499999999999886, 5.016499999999999737 ) ) ;
#3750=ORIENTED_EDGE ( 'NONE', *, *, #4875, .T. ) ;
#3763=ORIENTED_EDGE ( 'NONE', *, *, #25627, .F. ) ;
#3770=CARTESIAN_POINT ( 'NONE',  ( -5.177913976931285411, 57.14999999999999858, -5.372100000000001430 ) ) ;
#3776=EDGE_CURVE ( 'NONE', #5931, #35130, #2000, .T. ) ;
#3806=ADVANCED_FACE ( 'NONE', ( #24288 ), #10828, .F. ) ;
#3815=CARTESIAN_POINT ( 'NONE',  ( -14.50851225146815437, 78.09971119798315442, 5.392902600000138769 ) ) ;
#3832=ORIENTED_EDGE ( 'NONE', *, *, #38059, .F. ) ;
#3871=DIRECTION ( 'NONE',  ( 0.1469470846586743706, 9.335746474409589170E-17, 0.9891443546370348727 ) ) ;
#3878=CARTESIAN_POINT ( 'NONE',  ( 12.16475753114682767, 55.74362973025085211, 5.016499999999999737 ) ) ;
#3888=AXIS2_PLACEMENT_3D ( 'NONE', #31131, #1968, #18334 ) ;
#3891=CARTESIAN_POINT ( 'NONE',  ( -9.925711944554160837, 78.55658865046541450, -5.016499999999999737 ) ) ;
#3896=VERTEX_POINT ( 'NONE', #20040 ) ;
#3897=CARTESIAN_POINT ( 'NONE',  ( 5.177913976931216133, 53.58606249999999704, 5.372100000000000541 ) ) ;
#3900=CARTESIAN_POINT ( 'NONE',  ( -7.213960532363675959, 86.35999999999998522, 1.904999999999995364 ) ) ;
#3906=ORIENTED_EDGE ( 'NONE', *, *, #23278, .T. ) ;
#3908=VECTOR ( 'NONE', #38448, 1000.000000000000114 ) ;
#3915=CARTESIAN_POINT ( 'NONE',  ( 10.28897677580358128, 56.51500000000000057, 4.381499999999999950 ) ) ;
#3931=AXIS2_PLACEMENT_3D ( 'NONE', #29157, #12969, #25962 ) ;
#3936=CARTESIAN_POINT ( 'NONE',  ( -12.21488373879589240, 17.14500000000000313, -5.016499999999999737 ) ) ;
#3939=CARTESIAN_POINT ( 'NONE',  ( -5.706177858045075268, 56.51500000000000057, 5.041924731713889329 ) ) ;
#3940=CARTESIAN_POINT ( 'NONE',  ( -14.50851225146815615, 78.09971119798315442, -1.904999999999999583 ) ) ;
#3971=EDGE_CURVE ( 'NONE', #11659, #38242, #34652, .T. ) ;
#3994=EDGE_LOOP ( 'NONE', ( #26849, #22411, #31121, #13999 ) ) ;
#4001=CARTESIAN_POINT ( 'NONE',  ( -7.126949251439574695, 78.78385021288468693, -2.234499184491881785 ) ) ;
#4003=ORIENTED_EDGE ( 'NONE', *, *, #9224, .T. ) ;
#4019=ORIENTED_EDGE ( 'NONE', *, *, #6327, .F. ) ;
#4024=VERTEX_POINT ( 'NONE', #34730 ) ;
#4026=FACE_BOUND ( 'NONE', #29457, .T. ) ;
#4045=EDGE_CURVE ( 'NONE', #14016, #31005, #4752, .T. ) ;
#4053=CARTESIAN_POINT ( 'NONE',  ( 14.39766717389552220, 60.02151067229126369, 1.904999999999990923 ) ) ;
#4055=B_SPLINE_CURVE_WITH_KNOTS ( 'NONE', 3,
 ( #36196, #16146, #22737, #7017, #12191, #29148, #3396, #16362, #29368, #3614, #35562, #10191, #39388, #19985, #33002, #29795 ),
 .UNSPECIFIED., .F., .F.,
 ( 4, 2, 2, 2, 2, 2, 2, 4 ),
 ( 0.000000000000000000, 0.2499999999999863998, 0.3749999999999810152, 0.4374999999999812372, 0.4687499999999821809, 0.4999999999999831246, 0.7499999999999915623, 1.000000000000000000 ),
 .UNSPECIFIED. ) ;
#4058=EDGE_CURVE ( 'NONE', #11710, #42131, #8132, .T. ) ;
#4091=B_SPLINE_CURVE_WITH_KNOTS ( 'NONE', 3,
 ( #15674, #12908, #29528, #28678, #19084, #32087 ),
 .UNSPECIFIED., .F., .F.,
 ( 4, 2, 4 ),
 ( 0.07978617534960311120, 0.5398930876748015972, 1.000000000000000000 ),
 .UNSPECIFIED. ) ;
#4093=ORIENTED_EDGE ( 'NONE', *, *, #29178, .T. ) ;
#4097=CARTESIAN_POINT ( 'NONE',  ( 14.73199999999999754, 12.70000000000000107, 0.000000000000000000 ) ) ;
#4098=CARTESIAN_POINT ( 'NONE',  ( -10.79307885933853761, 57.10041794475097277, -5.016499999999999737 ) ) ;
#4106=VECTOR ( 'NONE', #12594, 1000.000000000000000 ) ;
#4113=EDGE_CURVE ( 'NONE', #1544, #29870, #2153, .T. ) ;
#4146=CARTESIAN_POINT ( 'NONE',  ( -6.059261036834497460, 77.01756250000002524, 5.016499999999999737 ) ) ;
#4155=CARTESIAN_POINT ( 'NONE',  ( 11.58677707360137532, 17.14499999999999957, 4.474811398758258285 ) ) ;
#4179=DIRECTION ( 'NONE',  ( 1.224646799147353207E-16, -1.179012811983454535E-32, 1.000000000000000000 ) ) ;
#4183=( BOUNDED_CURVE ( )  B_SPLINE_CURVE ( 3, ( #268, #2834, #22798, #22379 ),
 .UNSPECIFIED., .F., .T. ) 
 B_SPLINE_CURVE_WITH_KNOTS ( ( 4, 4 ),
 ( 1.570796326794897446, 3.141592653589792672 ),
 .UNSPECIFIED. ) 
 CURVE ( )  GEOMETRIC_REPRESENTATION_ITEM ( )  RATIONAL_B_SPLINE_CURVE ( ( 1.000000000000000000, 0.8047378541243652705, 0.8047378541243652705, 1.000000000000000000 ) ) 
 REPRESENTATION_ITEM ( '' )  );
#4186=VECTOR ( 'NONE', #29664, 1000.000000000000000 ) ;
#4208=CARTESIAN_POINT ( 'NONE',  ( -5.177913976931298734, 78.94499979771843812, -5.372100000000003206 ) ) ;
#4209=AXIS2_PLACEMENT_3D ( 'NONE', #17944, #37548, #39927 ) ;
#4214=ADVANCED_FACE ( 'NONE', ( #31949 ), #32794, .F. ) ;
#4217=DIRECTION ( 'NONE',  ( 0.1469470846586743984, 9.335746474409589170E-17, 0.9891443546370349837 ) ) ;
#4228=ORIENTED_EDGE ( 'NONE', *, *, #36531, .T. ) ;
#4244=CARTESIAN_POINT ( 'NONE',  ( -14.39766717389551864, 60.87500489999898434, -1.904999999999999583 ) ) ;
#4269=FACE_OUTER_BOUND ( 'NONE', #40486, .T. ) ;
#4274=AXIS2_PLACEMENT_3D ( 'NONE', #25349, #34731, #41126 ) ;
#4276=ORIENTED_EDGE ( 'NONE', *, *, #30098, .T. ) ;
#4294=DIRECTION ( 'NONE',  ( 0.000000000000000000, 1.000000000000000000, 0.000000000000000000 ) ) ;
#4297=EDGE_CURVE ( 'NONE', #5344, #4652, #5545, .T. ) ;
#4300=ADVANCED_FACE ( 'NONE', ( #28750 ), #41763, .T. ) ;
#4302=CARTESIAN_POINT ( 'NONE',  ( 11.47253659098475076, 56.76836532675937974, 5.016499999999999737 ) ) ;
#4305=VERTEX_POINT ( 'NONE', #16156 ) ;
#4309=CARTESIAN_POINT ( 'NONE',  ( -5.600204413207901410, 78.91171765783740000, 5.075433163388495039 ) ) ;
#4319=EDGE_CURVE ( 'NONE', #21156, #35348, #38351, .T. ) ;
#4321=CARTESIAN_POINT ( 'NONE',  ( -5.348924234571056147, 56.51499999999999346, 4.492130288940740179 ) ) ;
#4331=FACE_OUTER_BOUND ( 'NONE', #8085, .T. ) ;
#4333=AXIS2_PLACEMENT_3D ( 'NONE', #2314, #27644, #40863 ) ;
#4344=CARTESIAN_POINT ( 'NONE',  ( 10.28897677580358128, 56.51500000000000057, -4.381500000000000838 ) ) ;
#4345=VECTOR ( 'NONE', #40855, 1000.000000000000227 ) ;
#4350=EDGE_CURVE ( 'NONE', #38485, #39783, #9168, .T. ) ;
#4362=CARTESIAN_POINT ( 'NONE',  ( -5.115576404396798615, 56.51500000000000767, 4.603576161448844850 ) ) ;
#4382=CARTESIAN_POINT ( 'NONE',  ( 6.059261036834406866, 57.14999999999999858, 5.016499999999999737 ) ) ;
#4383=DIRECTION ( 'NONE',  ( 1.000000000000000000, 6.353134868986659519E-16, 0.000000000000000000 ) ) ;
#4398=ORIENTED_EDGE ( 'NONE', *, *, #16689, .T. ) ;
#4407=DIRECTION ( 'NONE',  ( -0.1728608224830406603, -1.098208118798718614E-16, -0.9849462604886047856 ) ) ;
#4416=ORIENTED_EDGE ( 'NONE', *, *, #6379, .F. ) ;
#4420=ORIENTED_EDGE ( 'NONE', *, *, #27782, .F. ) ;
#4425=DIRECTION ( 'NONE',  ( -1.000000000000000000, -6.353134868986659519E-16, 0.000000000000000000 ) ) ;
#4432=VERTEX_POINT ( 'NONE', #40039 ) ;
#4440=ORIENTED_EDGE ( 'NONE', *, *, #30050, .F. ) ;
#4453=FACE_OUTER_BOUND ( 'NONE', #29240, .T. ) ;
#4456=CARTESIAN_POINT ( 'NONE',  ( -5.486567272856878414E-14, 86.35999999999998522, 0.000000000000000000 ) ) ;
#4478=CARTESIAN_POINT ( 'NONE',  ( 5.305748947172191698, 88.73331249999999670, -5.247078976224250013 ) ) ;
#4484=ORIENTED_EDGE ( 'NONE', *, *, #4501, .F. ) ;
#4497=VERTEX_POINT ( 'NONE', #14229 ) ;
#4501=EDGE_CURVE ( 'NONE', #39783, #26876, #31229, .T. ) ;
#4505=CARTESIAN_POINT ( 'NONE',  ( 1.222676017494593648E-15, 12.70000000000000284, 0.000000000000000000 ) ) ;
#4514=DIRECTION ( 'NONE',  ( -1.000000000000000000, 0.000000000000000000, 0.000000000000000000 ) ) ;
#4515=FACE_OUTER_BOUND ( 'NONE', #30146, .T. ) ;
#4530=VERTEX_POINT ( 'NONE', #23170 ) ;
#4531=ORIENTED_EDGE ( 'NONE', *, *, #40973, .T. ) ;
#4540=CARTESIAN_POINT ( 'NONE',  ( 13.85159022459153988, 12.96416000000000146, 5.016499999999999737 ) ) ;
#4543=CIRCLE ( 'NONE', #27646, 7.461249999999999716 ) ;
#4595=VECTOR ( 'NONE', #25304, 1000.000000000000114 ) ;
#4596=EDGE_CURVE ( 'NONE', #5970, #33026, #37867, .T. ) ;
#4603=EDGE_CURVE ( 'NONE', #24258, #10259, #8293, .T. ) ;
#4629=DIRECTION ( 'NONE',  ( -1.000000000000000000, -6.353134868986659519E-16, 0.000000000000000000 ) ) ;
#4635=FACE_OUTER_BOUND ( 'NONE', #37201, .T. ) ;
#4644=ADVANCED_FACE ( 'NONE', ( #14853 ), #19824, .T. ) ;
#4652=VERTEX_POINT ( 'NONE', #11450 ) ;
#4654=PLANE ( 'NONE',  #33813 ) ;
#4655=LINE ( 'NONE', #39588, #19137 ) ;
#4660=CYLINDRICAL_SURFACE ( 'NONE', #21938, 16.60960244842765832 ) ;
#4662=DIRECTION ( 'NONE',  ( 0.000000000000000000, 0.000000000000000000, 1.000000000000000000 ) ) ;
#4683=LINE ( 'NONE', #17640, #17428 ) ;
#4685=CIRCLE ( 'NONE', #5385, 6.349999999999999645 ) ;
#4703=ORIENTED_EDGE ( 'NONE', *, *, #22711, .F. ) ;
#4713=CARTESIAN_POINT ( 'NONE',  ( -5.348924234571052594, 56.51499999999999346, -4.492130288940743732 ) ) ;
#4715=AXIS2_PLACEMENT_3D ( 'NONE', #25289, #37440, #5925 ) ;
#4744=ORIENTED_EDGE ( 'NONE', *, *, #13947, .T. ) ;
#4752=CIRCLE ( 'NONE', #28528, 12.69999999999999751 ) ;
#4755=EDGE_LOOP ( 'NONE', ( #40689, #38715, #8803, #166, #26044, #3509 ) ) ;
#4761=CARTESIAN_POINT ( 'NONE',  ( 11.48503488083538926, 55.92196062030127024, -5.016500000000110759 ) ) ;
#4772=AXIS2_PLACEMENT_3D ( 'NONE', #12478, #5465, #1848 ) ;
#4781=CARTESIAN_POINT ( 'NONE',  ( -5.322311914403968558, 56.51500000000043400, 5.239113282919425352 ) ) ;
#4815=LINE ( 'NONE', #31185, #6312 ) ;
#4823=AXIS2_PLACEMENT_3D ( 'NONE', #40329, #27316, #34139 ) ;
#4828=ORIENTED_EDGE ( 'NONE', *, *, #30807, .F. ) ;
#4840=ORIENTED_EDGE ( 'NONE', *, *, #29765, .F. ) ;
#4845=ORIENTED_EDGE ( 'NONE', *, *, #10234, .T. ) ;
#4854=CIRCLE ( 'NONE', #10926, 7.461249999999999716 ) ;
#4855=ORIENTED_EDGE ( 'NONE', *, *, #738, .T. ) ;
#4858=AXIS2_PLACEMENT_3D ( 'NONE', #41737, #21273, #2561 ) ;
#4862=VERTEX_POINT ( 'NONE', #2141 ) ;
#4874=AXIS2_PLACEMENT_3D ( 'NONE', #24102, #18330, #1964 ) ;
#4875=EDGE_CURVE ( 'NONE', #32761, #22572, #32771, .T. ) ;
#4898=CARTESIAN_POINT ( 'NONE',  ( -6.350000000000053824, 83.56599999999998829, 7.776507174585703010E-16 ) ) ;
#4914=VECTOR ( 'NONE', #23918, 1000.000000000000000 ) ;
#4924=CARTESIAN_POINT ( 'NONE',  ( 13.85159022459153988, 12.96416000000000146, 5.016499999999999737 ) ) ;
#4937=CARTESIAN_POINT ( 'NONE',  ( 1.406077420118782567E-15, 14.60500000000000220, 0.000000000000000000 ) ) ;
#4948=VERTEX_POINT ( 'NONE', #18930 ) ;
#4950=ORIENTED_EDGE ( 'NONE', *, *, #25311, .T. ) ;
#4964=CARTESIAN_POINT ( 'NONE',  ( 12.21488373879589240, 55.24500000000000455, -5.016500000000000625 ) ) ;
#4965=CIRCLE ( 'NONE', #34872, 0.6349999999999984546 ) ;
#4976=EDGE_CURVE ( 'NONE', #19939, #6797, #18714, .T. ) ;
#4977=AXIS2_PLACEMENT_3D ( 'NONE', #37645, #18450, #15046 ) ;
#4981=CARTESIAN_POINT ( 'NONE',  ( -6.059261036834487690, 71.63300248836198136, -5.016499999999999737 ) ) ;
#4987=DIRECTION ( 'NONE',  ( -1.000000000000000000, 0.000000000000000000, 0.000000000000000000 ) ) ;
#5004=CARTESIAN_POINT ( 'NONE',  ( 5.936184715466450434, 56.51500000000000057, 4.381499802638942676 ) ) ;
#5011=EDGE_CURVE ( 'NONE', #18746, #4497, #25280, .T. ) ;
#5021=VECTOR ( 'NONE', #11832, 1000.000000000000000 ) ;
#5023=EDGE_CURVE ( 'NONE', #33803, #38620, #16421, .T. ) ;
#5064=EDGE_CURVE ( 'NONE', #32592, #5970, #30425, .T. ) ;
#5067=EDGE_CURVE ( 'NONE', #22768, #29525, #23905, .T. ) ;
#5072=CARTESIAN_POINT ( 'NONE',  ( 5.348924234570989533, 56.51499999999999346, 4.492130288940735738 ) ) ;
#5073=VERTEX_POINT ( 'NONE', #24909 ) ;
#5089=DIRECTION ( 'NONE',  ( -1.000000000000000000, -6.353134868986659519E-16, 0.000000000000000000 ) ) ;
#5135=CARTESIAN_POINT ( 'NONE',  ( 6.059261036834394432, 71.63300248836199557, -5.016499999999999737 ) ) ;
#5138=CARTESIAN_POINT ( 'NONE',  ( 8.947566919452587848E-16, 9.293884745518887769, 0.000000000000000000 ) ) ;
#5156=ORIENTED_EDGE ( 'NONE', *, *, #18565, .T. ) ;
#5163=ORIENTED_EDGE ( 'NONE', *, *, #4297, .F. ) ;
#5167=LINE ( 'NONE', #5586, #15722 ) ;
#5168=ADVANCED_FACE ( 'NONE', ( #37909 ), #1935, .F. ) ;
#5173=EDGE_CURVE ( 'NONE', #117, #4432, #38222, .T. ) ;
#5179=CARTESIAN_POINT ( 'NONE',  ( 10.62867326514809463, 56.48194529650093187, -4.405924061720181584 ) ) ;
#5192=CARTESIAN_POINT ( 'NONE',  ( -12.21488373879589240, 17.14499999999999957, 4.381499999999999950 ) ) ;
#5233=TOROIDAL_SURFACE ( 'NONE', #3184, 6.985000000000000320, 0.6350000000000000089 ) ;
#5234=DIRECTION ( 'NONE',  ( -1.000000000000000000, 0.000000000000000000, 0.000000000000000000 ) ) ;
#5235=ORIENTED_EDGE ( 'NONE', *, *, #26947, .T. ) ;
#5259=CARTESIAN_POINT ( 'NONE',  ( 1.589478822742971486E-15, 16.51000000000000156, 0.000000000000000000 ) ) ;
#5260=ORIENTED_EDGE ( 'NONE', *, *, #10766, .T. ) ;
#5272=ORIENTED_EDGE ( 'NONE', *, *, #18338, .T. ) ;
#5290=DIRECTION ( 'NONE',  ( -0.9891443546370349837, 0.000000000000000000, 0.1469470846586743706 ) ) ;
#5297=ORIENTED_EDGE ( 'NONE', *, *, #23821, .T. ) ;
#5309=CARTESIAN_POINT ( 'NONE',  ( 7.019433301159567762, 78.79326733250422876, -2.552382320839209573 ) ) ;
#5330=ORIENTED_EDGE ( 'NONE', *, *, #40453, .T. ) ;
#5332=CARTESIAN_POINT ( 'NONE',  ( -5.664977208693890098, 57.14999999999999147, 5.033228321271210781 ) ) ;
#5341=CARTESIAN_POINT ( 'NONE',  ( -18.35410564743290607, 77.35382415001784295, 1.904999999999988480 ) ) ;
#5343=ORIENTED_EDGE ( 'NONE', *, *, #10441, .T. ) ;
#5344=VERTEX_POINT ( 'NONE', #32559 ) ;
#5350=CARTESIAN_POINT ( 'NONE',  ( -11.32678463655042478, 56.02547433970777035, -4.456118031212342068 ) ) ;
#5370=ORIENTED_EDGE ( 'NONE', *, *, #19801, .F. ) ;
#5375=CARTESIAN_POINT ( 'NONE',  ( 13.46199999999999797, 12.17394877578616708, 0.000000000000000000 ) ) ;
#5384=DIRECTION ( 'NONE',  ( -1.000000000000000000, 9.627370216492862708E-17, 0.000000000000000000 ) ) ;
#5385=AXIS2_PLACEMENT_3D ( 'NONE', #20306, #23932, #16493 ) ;
#5399=CARTESIAN_POINT ( 'NONE',  ( -5.382937502775954980E-14, 83.56599999999998829, -1.904999999999999805 ) ) ;
#5403=DIRECTION ( 'NONE',  ( 0.000000000000000000, -0.000000000000000000, 1.000000000000000000 ) ) ;
#5409=VECTOR ( 'NONE', #6805, 1000.000000000000000 ) ;
#5419=VERTEX_POINT ( 'NONE', #13180 ) ;
#5440=DIRECTION ( 'NONE',  ( -1.000000000000000000, -6.353134868986659519E-16, -0.000000000000000000 ) ) ;
#5452=ORIENTED_EDGE ( 'NONE', *, *, #23772, .T. ) ;
#5457=CARTESIAN_POINT ( 'NONE',  ( 5.177913976931196594, 78.94499979771845233, -5.372100000000001430 ) ) ;
#5465=DIRECTION ( 'NONE',  ( -5.463695987328526437E-16, 1.000000000000000000, 1.672774450599033775E-31 ) ) ;
#5466=ORIENTED_EDGE ( 'NONE', *, *, #25402, .F. ) ;
#5484=DIRECTION ( 'NONE',  ( 0.000000000000000000, 1.000000000000000000, 0.000000000000000000 ) ) ;
#5492=CARTESIAN_POINT ( 'NONE',  ( 5.353961914031110325, 56.51499999999804658, -5.213928161110970905 ) ) ;
#5501=ORIENTED_EDGE ( 'NONE', *, *, #13894, .F. ) ;
#5504=DIRECTION ( 'NONE',  ( -0.1469470846586743706, 0.000000000000000000, -0.9891443546370348727 ) ) ;
#5513=DIRECTION ( 'NONE',  ( 6.146657985744592735E-16, 3.905054717696927382E-31, 1.000000000000000000 ) ) ;
#5521=VECTOR ( 'NONE', #18287, 1000.000000000000000 ) ;
#5538=CARTESIAN_POINT ( 'NONE',  ( -5.241362157049126225, 57.14999999999999147, 5.310945289804169356 ) ) ;
#5543=CARTESIAN_POINT ( 'NONE',  ( -4.781543117819943234, 56.51500000000003610, -4.872198453344445568 ) ) ;
#5545=B_SPLINE_CURVE_WITH_KNOTS ( 'NONE', 3,
 ( #26177, #38763, #3193, #25756, #29378, #431 ),
 .UNSPECIFIED., .F., .F.,
 ( 4, 2, 4 ),
 ( 0.000000000000000000, 0.5000000000000000000, 1.000000000000000000 ),
 .UNSPECIFIED. ) ;
#5558=LINE ( 'NONE', #27285, #29085 ) ;
#5581=DIRECTION ( 'NONE',  ( -0.1715592850456333085, -0.1224830539174543292, 0.9775302108976914317 ) ) ;
#5586=CARTESIAN_POINT ( 'NONE',  ( 6.057513928997550146, 86.35999999999998522, -1.904999999999999805 ) ) ;
#5599=LINE ( 'NONE', #24957, #36807 ) ;
#5618=DIRECTION ( 'NONE',  ( -1.000000000000000000, 0.000000000000000000, 0.000000000000000000 ) ) ;
#5619=DIRECTION ( 'NONE',  ( -0.000000000000000000, -0.000000000000000000, -1.000000000000000000 ) ) ;
#5622=ORIENTED_EDGE ( 'NONE', *, *, #38069, .F. ) ;
#5634=ORIENTED_EDGE ( 'NONE', *, *, #2083, .T. ) ;
#5644=B_SPLINE_CURVE_WITH_KNOTS ( 'NONE', 3,
 ( #21446, #34476, #12096, #21872, #25084, #41504, #12310, #5309, #31476, #38091 ),
 .UNSPECIFIED., .F., .F.,
 ( 4, 2, 2, 2, 4 ),
 ( -0.0004895961982421361599, 0.0005229314014804232590, 0.001535459001202982678, 0.002547986600925542314, 0.003560514200648101299 ),
 .UNSPECIFIED. ) ;
#5665=FACE_OUTER_BOUND ( 'NONE', #37347, .T. ) ;
#5677=CARTESIAN_POINT ( 'NONE',  ( 5.525651935317158703, 78.91763798174282840, -5.107334513333023018 ) ) ;
#5705=AXIS2_PLACEMENT_3D ( 'NONE', #23947, #4179, #27364 ) ;
#5709=CARTESIAN_POINT ( 'NONE',  ( 14.60500000000000043, 71.11999999999999034, 5.016499999999999737 ) ) ;
#5715=CARTESIAN_POINT ( 'NONE',  ( -5.638141748396392039, 57.15000000000040359, 5.060111600445807767 ) ) ;
#5721=AXIS2_PLACEMENT_3D ( 'NONE', #37398, #18417, #2266 ) ;
#5725=VERTEX_POINT ( 'NONE', #3936 ) ;
#5735=CARTESIAN_POINT ( 'NONE',  ( -20.83467972660109524, 65.95194780259438971, -1.904999999999999583 ) ) ;
#5736=CARTESIAN_POINT ( 'NONE',  ( 5.511339492712161281, 56.51499999999996504, 5.111277471823914453 ) ) ;
#5741=AXIS2_PLACEMENT_3D ( 'NONE', #24274, #8098, #17466 ) ;
#5748=EDGE_LOOP ( 'NONE', ( #2074, #21257 ) ) ;
#5754=CARTESIAN_POINT ( 'NONE',  ( -14.73199999999999932, 12.96416000000000146, 0.000000000000000000 ) ) ;
#5755=VECTOR ( 'NONE', #4383, 1000.000000000000000 ) ;
#5775=LINE ( 'NONE', #31109, #26003 ) ;
#5778=CARTESIAN_POINT ( 'NONE',  ( -5.153324091238889793, 56.51694919289756314, 4.640537933326888798 ) ) ;
#5790=ORIENTED_EDGE ( 'NONE', *, *, #21638, .T. ) ;
#5793=( NAMED_UNIT ( * ) PLANE_ANGLE_UNIT ( ) SI_UNIT ( $, .RADIAN. ) );
#5795=DIRECTION ( 'NONE',  ( 1.000000000000000000, 6.353134868986659519E-16, 0.000000000000000000 ) ) ;
#5807=DIRECTION ( 'NONE',  ( 0.1469470846586743706, 0.000000000000000000, 0.9891443546370348727 ) ) ;
#5860=DIRECTION ( 'NONE',  ( 0.000000000000000000, 1.000000000000000000, 0.000000000000000000 ) ) ;
#5870=CARTESIAN_POINT ( 'NONE',  ( -6.059261036834497460, 88.73331249999999670, -5.016499999999999737 ) ) ;
#5873=VERTEX_POINT ( 'NONE', #40133 ) ;
#5885=ADVANCED_FACE ( 'NONE', ( #39641 ), #1089, .T. ) ;
#5917=CARTESIAN_POINT ( 'NONE',  ( 5.450166374333662134, 56.51500000000003610, -4.451212169035211552 ) ) ;
#5925=DIRECTION ( 'NONE',  ( -1.000000000000000000, 0.000000000000000000, 0.000000000000000000 ) ) ;
#5930=EDGE_CURVE ( 'NONE', #17444, #16646, #7072, .T. ) ;
#5931=VERTEX_POINT ( 'NONE', #10023 ) ;
#5936=AXIS2_PLACEMENT_3D ( 'NONE', #23220, #36886, #14072 ) ;
#5939=ADVANCED_FACE ( 'NONE', ( #17040 ), #7686, .F. ) ;
#5960=CARTESIAN_POINT ( 'NONE',  ( 18.32410244842765934, 8.844871939465424049, 2.244055341071511024E-15 ) ) ;
#5964=CARTESIAN_POINT ( 'NONE',  ( -15.36699999999999378, 12.96302561210691984, 0.000000000000000000 ) ) ;
#5970=VERTEX_POINT ( 'NONE', #13227 ) ;
#5972=CARTESIAN_POINT ( 'NONE',  ( 14.73199999999999754, 61.59499999999999886, 5.016499999999999737 ) ) ;
#5989=ORIENTED_EDGE ( 'NONE', *, *, #23477, .F. ) ;
#5998=CARTESIAN_POINT ( 'NONE',  ( -13.46199999999999442, 12.17394877578617063, 1.841354584184931751E-15 ) ) ;
#6014=STYLED_ITEM ( 'NONE', ( #11741 ), #21408 ) ;
#6018=CARTESIAN_POINT ( 'NONE',  ( -5.451267667241070720E-14, 85.80437499999999318, 0.000000000000000000 ) ) ;
#6053=CIRCLE ( 'NONE', #35292, 6.350000000000004974 ) ;
#6059=ORIENTED_EDGE ( 'NONE', *, *, #13894, .T. ) ;
#6077=CARTESIAN_POINT ( 'NONE',  ( -5.965356522962928842, 53.58606249999999704, -5.016499999999999737 ) ) ;
#6084=ORIENTED_EDGE ( 'NONE', *, *, #23404, .F. ) ;
#6092=LINE ( 'NONE', #41666, #1308 ) ;
#6109=EDGE_CURVE ( 'NONE', #13560, #20581, #40109, .T. ) ;
#6116=ORIENTED_EDGE ( 'NONE', *, *, #24581, .T. ) ;
#6127=DIRECTION ( 'NONE',  ( -1.000000000000000000, 0.000000000000000000, -0.000000000000000000 ) ) ;
#6135=CARTESIAN_POINT ( 'NONE',  ( 13.85159022459153988, 59.63164443796365077, 5.016499999999999737 ) ) ;
#6140=DIRECTION ( 'NONE',  ( -0.000000000000000000, -0.000000000000000000, -1.000000000000000000 ) ) ;
#6159=ORIENTED_EDGE ( 'NONE', *, *, #30069, .T. ) ;
#6167=CARTESIAN_POINT ( 'NONE',  ( 5.266289895157169814E-14, 83.56599999999998829, 1.904999999999999805 ) ) ;
#6176=ORIENTED_EDGE ( 'NONE', *, *, #3424, .F. ) ;
#6185=DIRECTION ( 'NONE',  ( 1.000000000000000000, 6.353134868986659519E-16, 0.000000000000000000 ) ) ;
#6186=LINE ( 'NONE', #19361, #18516 ) ;
#6189=CARTESIAN_POINT ( 'NONE',  ( -13.46199999999999442, 12.17394877578617063, 1.648619521012166368E-15 ) ) ;
#6210=CARTESIAN_POINT ( 'NONE',  ( -18.35410564743290607, 77.35382415001784295, 1.904999999999988480 ) ) ;
#6225=DIRECTION ( 'NONE',  ( 9.627370216492862708E-17, 1.000000000000000000, -0.000000000000000000 ) ) ;
#6236=FACE_OUTER_BOUND ( 'NONE', #2164, .T. ) ;
#6237=FACE_OUTER_BOUND ( 'NONE', #22954, .T. ) ;
#6243=ORIENTED_EDGE ( 'NONE', *, *, #14042, .F. ) ;
#6245=AXIS2_PLACEMENT_3D ( 'NONE', #16132, #42153, #195 ) ;
#6271=LINE ( 'NONE', #16248, #16510 ) ;
#6282=CARTESIAN_POINT ( 'NONE',  ( -5.965356522962950159, 88.73331249999999670, -5.016499999999999737 ) ) ;
#6286=EDGE_LOOP ( 'NONE', ( #8296, #31096, #31369, #20347 ) ) ;
#6294=CARTESIAN_POINT ( 'NONE',  ( 5.809014734623085374, 78.89492211486508211, -5.027281507146220463 ) ) ;
#6302=CARTESIAN_POINT ( 'NONE',  ( 12.21488373879589240, 12.96416000000000146, 4.381499999999999950 ) ) ;
#6312=VECTOR ( 'NONE', #1616, 1000.000000000000000 ) ;
#6319=EDGE_LOOP ( 'NONE', ( #11536, #38368, #8509, #24109 ) ) ;
#6327=EDGE_CURVE ( 'NONE', #1883, #8736, #26921, .T. ) ;
#6334=VERTEX_POINT ( 'NONE', #36910 ) ;
#6346=LINE ( 'NONE', #35950, #30598 ) ;
#6364=CARTESIAN_POINT ( 'NONE',  ( 18.35410564743290962, 77.35382415001784295, 5.392902600000138769 ) ) ;
#6379=EDGE_CURVE ( 'NONE', #22830, #2471, #27007, .T. ) ;
#6381=ORIENTED_EDGE ( 'NONE', *, *, #363, .F. ) ;
#6404=EDGE_CURVE ( 'NONE', #10059, #25746, #24513, .T. ) ;
#6407=VERTEX_POINT ( 'NONE', #8980 ) ;
#6421=CARTESIAN_POINT ( 'NONE',  ( 14.73199999999999932, 12.96416000000000146, 0.000000000000000000 ) ) ;
#6427=DIRECTION ( 'NONE',  ( 1.000000000000000000, -9.466894658874049451E-17, 0.000000000000000000 ) ) ;
#6428=CARTESIAN_POINT ( 'NONE',  ( 12.69999999999999929, 14.60500000000000043, 0.000000000000000000 ) ) ;
#6440=DIRECTION ( 'NONE',  ( -1.000000000000000000, 0.000000000000000000, 0.000000000000000000 ) ) ;
#6446=EDGE_CURVE ( 'NONE', #24827, #25703, #31076, .T. ) ;
#6448=CYLINDRICAL_SURFACE ( 'NONE', #28786, 0.6349999999999966782 ) ;
#6471=CARTESIAN_POINT ( 'NONE',  ( 18.35410564743290962, 77.35382415001784295, -1.904999999999999583 ) ) ;
#6502=CARTESIAN_POINT ( 'NONE',  ( 14.39766717389552220, 60.02151067229126369, 1.904999999999990923 ) ) ;
#6508=VERTEX_POINT ( 'NONE', #21734 ) ;
#6521=FACE_OUTER_BOUND ( 'NONE', #23576, .T. ) ;
#6545=ADVANCED_FACE ( 'NONE', ( #24735 ), #37737, .T. ) ;
#6560=EDGE_LOOP ( 'NONE', ( #35466, #6968, #21840, #38731 ) ) ;
#6563=AXIS2_PLACEMENT_3D ( 'NONE', #9056, #22021, #38659 ) ;
#6568=ORIENTED_EDGE ( 'NONE', *, *, #26593, .T. ) ;
#6576=CARTESIAN_POINT ( 'NONE',  ( -5.638212235186761845, 57.15000000000000568, -5.060089761242226203 ) ) ;
#6579=CARTESIAN_POINT ( 'NONE',  ( 2.407412430484044816E-32, 1.626303258728256651E-15, 0.000000000000000000 ) ) ;
#6632=LINE ( 'NONE', #36237, #40900 ) ;
#6639=EDGE_CURVE ( 'NONE', #16922, #6508, #18546, .T. ) ;
#6653=FACE_OUTER_BOUND ( 'NONE', #23340, .T. ) ;
#6657=VECTOR ( 'NONE', #12141, 1000.000000000000000 ) ;
#6659=CARTESIAN_POINT ( 'NONE',  ( 5.664977208693799504, 88.73331249999999670, 5.033228321271210781 ) ) ;
#6670=CARTESIAN_POINT ( 'NONE',  ( 0.000000000000000000, 0.000000000000000000, 0.000000000000000000 ) ) ;
#6683=CARTESIAN_POINT ( 'NONE',  ( 8.515285667870289099E-16, 8.844871939465425825, 0.000000000000000000 ) ) ;
#6697=CARTESIAN_POINT ( 'NONE',  ( -5.177913976931305839, 88.73331249999998249, 5.372100000000000541 ) ) ;
#6708=PLANE ( 'NONE',  #30775 ) ;
#6719=ORIENTED_EDGE ( 'NONE', *, *, #34761, .T. ) ;
#6723=DIRECTION ( 'NONE',  ( -1.000000000000000000, -6.353134868986659519E-16, 0.000000000000000000 ) ) ;
#6742=VECTOR ( 'NONE', #39733, 1000.000000000000114 ) ;
#6748=CARTESIAN_POINT ( 'NONE',  ( -14.73199999999999754, 61.59499999999999886, 5.016499999999999737 ) ) ;
#6751=ORIENTED_EDGE ( 'NONE', *, *, #14101, .F. ) ;
#6756=CARTESIAN_POINT ( 'NONE',  ( 14.24929227862422820, 61.25037559889039329, 5.016500000000000625 ) ) ;
#6762=CARTESIAN_POINT ( 'NONE',  ( 16.87828382557106721, 17.14499999999999957, -5.016499999999999737 ) ) ;
#6788=CARTESIAN_POINT ( 'NONE',  ( -5.638212235253867277, 56.51500000000000767, -5.060089761408552711 ) ) ;
#6796=ORIENTED_EDGE ( 'NONE', *, *, #22369, .T. ) ;
#6797=VERTEX_POINT ( 'NONE', #6210 ) ;
#6804=CARTESIAN_POINT ( 'NONE',  ( 8.936628967501334841, 55.24500000000000455, 4.721553682181185430 ) ) ;
#6805=DIRECTION ( 'NONE',  ( 1.000000000000000000, -9.627370216492862708E-17, 0.000000000000000000 ) ) ;
#6808=SURFACE_SIDE_STYLE ('',( #12976 ) ) ;
#6840=CARTESIAN_POINT ( 'NONE',  ( 12.21488373879589240, 17.14499999999999957, -5.016499999999999737 ) ) ;
#6848=EDGE_CURVE ( 'NONE', #8022, #32592, #13222, .T. ) ;
#6859=DIRECTION ( 'NONE',  ( -0.000000000000000000, -1.000000000000000000, -0.000000000000000000 ) ) ;
#6867=LINE ( 'NONE', #3900, #24692 ) ;
#6873=EDGE_CURVE ( 'NONE', #32351, #38361, #482, .T. ) ;
#6879=PRODUCT_DEFINITION_SHAPE ( 'NONE', 'NONE',  #31572 ) ;
#6904=CARTESIAN_POINT ( 'NONE',  ( 6.608367952640213261, 78.82866613109550258, 3.480504251946402228 ) ) ;
#6911=CARTESIAN_POINT ( 'NONE',  ( -6.059261036834477920, 56.51499999999997925, 5.016500000000000625 ) ) ;
#6920=ORIENTED_EDGE ( 'NONE', *, *, #35461, .T. ) ;
#6928=CARTESIAN_POINT ( 'NONE',  ( 18.35410564743290607, 77.35382415001784295, 1.904999999999988480 ) ) ;
#6932=DIRECTION ( 'NONE',  ( 1.000000000000000000, -9.627370216492862708E-17, 0.000000000000000000 ) ) ;
#6937=CARTESIAN_POINT ( 'NONE',  ( 7.213960532367366341, 78.77618639008778700, 1.904999999999999583 ) ) ;
#6941=AXIS2_PLACEMENT_3D ( 'NONE', #5138, #18717, #31940 ) ;
#6955=DIRECTION ( 'NONE',  ( -1.000000000000000000, 0.000000000000000000, 0.000000000000000000 ) ) ;
#6963=CARTESIAN_POINT ( 'NONE',  ( -15.50061618130081165, 62.14374591690594940, -1.904999999999999583 ) ) ;
#6964=FACE_OUTER_BOUND ( 'NONE', #22805, .T. ) ;
#6968=ORIENTED_EDGE ( 'NONE', *, *, #25636, .T. ) ;
#6981=FACE_OUTER_BOUND ( 'NONE', #40190, .T. ) ;
#6993=FACE_OUTER_BOUND ( 'NONE', #33239, .T. ) ;
#7002=CARTESIAN_POINT ( 'NONE',  ( -18.35410564743290962, 77.35382415001784295, 1.904999999999988258 ) ) ;
#7017=CARTESIAN_POINT ( 'NONE',  ( -5.777868923222812647, 78.89722547516474549, -5.030779815616708284 ) ) ;
#7018=ORIENTED_EDGE ( 'NONE', *, *, #7400, .F. ) ;
#7024=CIRCLE ( 'NONE', #13821, 13.46199999999999442 ) ;
#7040=TOROIDAL_SURFACE ( 'NONE', #11759, 17.68910244842765778, 0.6350000000000000089 ) ;
#7060=AXIS2_PLACEMENT_3D ( 'NONE', #2918, #31872, #28674 ) ;
#7063=TOROIDAL_SURFACE ( 'NONE', #11124, 6.826249999999999929, 0.6350000000000000089 ) ;
#7065=CARTESIAN_POINT ( 'NONE',  ( 11.66725022231030628, 55.24499999999999744, 5.016500000000000625 ) ) ;
#7072=CIRCLE ( 'NONE', #13205, 0.6350000000000001199 ) ;
#7073=CARTESIAN_POINT ( 'NONE',  ( -5.767947771862510287, 78.89823565723088450, 5.032924692340702499 ) ) ;
#7074=CARTESIAN_POINT ( 'NONE',  ( -10.94257363143045936, 56.35470871607773091, -4.428493390991015133 ) ) ;
#7093=EDGE_CURVE ( 'NONE', #20396, #32690, #29404, .T. ) ;
#7095=ORIENTED_EDGE ( 'NONE', *, *, #30382, .F. ) ;
#7104=ORIENTED_EDGE ( 'NONE', *, *, #9655, .F. ) ;
#7117=TOROIDAL_SURFACE ( 'NONE', #2349, 6.985000000000000320, 0.6350000000000000089 ) ;
#7129=CARTESIAN_POINT ( 'NONE',  ( -5.860205464978564649, 56.51500000000000057, 5.019550312247363699 ) ) ;
#7134=ORIENTED_EDGE ( 'NONE', *, *, #27688, .T. ) ;
#7185=ORIENTED_EDGE ( 'NONE', *, *, #28499, .T. ) ;
#7194=ORIENTED_EDGE ( 'NONE', *, *, #24223, .T. ) ;
#7197=CARTESIAN_POINT ( 'NONE',  ( -13.85159022459153988, 59.63164443796365077, -5.016499999999999737 ) ) ;
#7203=CARTESIAN_POINT ( 'NONE',  ( 5.860279866612397193, 56.51500000000084611, 5.019549989587896555 ) ) ;
#7221=FACE_OUTER_BOUND ( 'NONE', #15518, .T. ) ;
#7268=CARTESIAN_POINT ( 'NONE',  ( 12.21488373879589240, 55.24500000000000455, 5.016499999999999737 ) ) ;
#7331=CYLINDRICAL_SURFACE ( 'NONE', #17121, 2.540000000000000480 ) ;
#7351=CARTESIAN_POINT ( 'NONE',  ( -18.35410564743290607, 77.35382415001784295, -1.904999999999999583 ) ) ;
#7352=LINE ( 'NONE', #1177, #22047 ) ;
#7391=CARTESIAN_POINT ( 'NONE',  ( -7.213960532367465817, 78.77618639008778700, -1.904999999999999583 ) ) ;
#7396=CARTESIAN_POINT ( 'NONE',  ( 13.34576682144454196, 17.14499999999997115, 5.016499999999998849 ) ) ;
#7400=EDGE_CURVE ( 'NONE', #22739, #15866, #40434, .T. ) ;
#7416=CARTESIAN_POINT ( 'NONE',  ( -3.590474171207809651E-14, 56.51499999999999346, 0.000000000000000000 ) ) ;
#7419=ORIENTED_EDGE ( 'NONE', *, *, #22679, .T. ) ;
#7426=DIRECTION ( 'NONE',  ( 6.353134868986659519E-16, -1.000000000000000000, 0.000000000000000000 ) ) ;
#7440=AXIS2_PLACEMENT_3D ( 'NONE', #16373, #32573, #32365 ) ;
#7456=CARTESIAN_POINT ( 'NONE',  ( 5.177913976931193041, 88.73331249999999670, -5.372100000000000541 ) ) ;
#7471=EDGE_CURVE ( 'NONE', #38361, #41795, #31923, .T. ) ;
#7485=CARTESIAN_POINT ( 'NONE',  ( 11.37822013471386207, 56.06794068206382775, 5.016500000000000625 ) ) ;
#7496=DIRECTION ( 'NONE',  ( 0.000000000000000000, 0.000000000000000000, -1.000000000000000000 ) ) ;
#7504=ORIENTED_EDGE ( 'NONE', *, *, #11013, .F. ) ;
#7509=EDGE_LOOP ( 'NONE', ( #14661, #32317 ) ) ;
#7535=ORIENTED_EDGE ( 'NONE', *, *, #8734, .T. ) ;
#7536=CARTESIAN_POINT ( 'NONE',  ( -12.69999999999999574, 14.60500000000000398, 1.555301434917138235E-15 ) ) ;
#7541=CARTESIAN_POINT ( 'NONE',  ( -5.256643466096560857, 56.51499999999957424, 5.296410793414254137 ) ) ;
#7548=CARTESIAN_POINT ( 'NONE',  ( -4.968812502051799918, 56.51947257897022325, 4.801689445547930646 ) ) ;
#7580=DIRECTION ( 'NONE',  ( 0.1728608224830406603, 1.098208118798718614E-16, 0.9849462604886047856 ) ) ;
#7589=CARTESIAN_POINT ( 'NONE',  ( 13.46199999999999619, 13.84300000000000175, 0.000000000000000000 ) ) ;
#7609=CARTESIAN_POINT ( 'NONE',  ( 9.638062024671789629, 56.51500000000000057, 4.786355703798467734E-15 ) ) ;
#7618=CIRCLE ( 'NONE', #36872, 6.905625000000000568 ) ;
#7622=ORIENTED_EDGE ( 'NONE', *, *, #26920, .T. ) ;
#7631=DIRECTION ( 'NONE',  ( -0.1469470846586743706, 1.414713986243376972E-17, 0.9891443546370348727 ) ) ;
#7646=ORIENTED_EDGE ( 'NONE', *, *, #33633, .T. ) ;
#7649=EDGE_CURVE ( 'NONE', #37617, #27765, #28104, .T. ) ;
#7663=CARTESIAN_POINT ( 'NONE',  ( 7.461249999999948201, 83.56599999999998829, 6.819232607250622208E-46 ) ) ;
#7665=CARTESIAN_POINT ( 'NONE',  ( 5.871452009091292723, 77.01756249999996840, -5.016499999999999737 ) ) ;
#7678=ORIENTED_EDGE ( 'NONE', *, *, #14926, .T. ) ;
#7685=ORIENTED_EDGE ( 'NONE', *, *, #33617, .F. ) ;
#7686=CYLINDRICAL_SURFACE ( 'NONE', #11825, 2.540000000000000480 ) ;
#7703=CARTESIAN_POINT ( 'NONE',  ( -5.477532837487763651, 78.92140300690499544, 5.132221182818779148 ) ) ;
#7704=CARTESIAN_POINT ( 'NONE',  ( 15.50061618130081165, 62.14374591690594940, 1.904999999999990035 ) ) ;
#7714=DIRECTION ( 'NONE',  ( -1.000000000000000000, -1.092739197465705287E-15, 0.000000000000000000 ) ) ;
#7731=ORIENTED_EDGE ( 'NONE', *, *, #29812, .F. ) ;
#7733=CARTESIAN_POINT ( 'NONE',  ( 11.82906070755469763, 56.41571150956137615, -5.016500000000000625 ) ) ;
#7753=CARTESIAN_POINT ( 'NONE',  ( -5.177913976931286300, 56.51500000000000057, 5.372100000000003206 ) ) ;
#7761=FACE_OUTER_BOUND ( 'NONE', #40766, .T. ) ;
#7774=ORIENTED_EDGE ( 'NONE', *, *, #16668, .T. ) ;
#7796=CARTESIAN_POINT ( 'NONE',  ( -13.11133394554952680, 57.78499999999998948, 9.234417301169688841 ) ) ;
#7806=ORIENTED_EDGE ( 'NONE', *, *, #37587, .F. ) ;
#7815=CARTESIAN_POINT ( 'NONE',  ( -5.423544988499506836, 78.92590603608628896, -5.135347845727594063 ) ) ;
#7820=CARTESIAN_POINT ( 'NONE',  ( -6.059261036834480585, 64.39150124418100063, 5.016499999999999737 ) ) ;
#7837=CARTESIAN_POINT ( 'NONE',  ( -10.41103689192127568, 56.51499999999998636, -5.203122797516516407 ) ) ;
#7847=FACE_OUTER_BOUND ( 'NONE', #11357, .T. ) ;
#7873=CARTESIAN_POINT ( 'NONE',  ( 5.664977208693799504, 77.01756249999996840, -5.033228321271210781 ) ) ;
#7879=ORIENTED_EDGE ( 'NONE', *, *, #29765, .T. ) ;
#7903=CIRCLE ( 'NONE', #36491, 0.6350000000000001199 ) ;
#7908=DIRECTION ( 'NONE',  ( 6.353134868986659519E-16, -1.000000000000000000, 0.000000000000000000 ) ) ;
#7918=CARTESIAN_POINT ( 'NONE',  ( 13.85159022459153988, 16.51000000000000156, -5.016499999999999737 ) ) ;
#7919=VERTEX_POINT ( 'NONE', #14826 ) ;
#7929=EDGE_CURVE ( 'NONE', #15919, #42038, #11856, .T. ) ;
#7930=CARTESIAN_POINT ( 'NONE',  ( -5.309060684617390516E-14, 83.56599999999998829, 0.000000000000000000 ) ) ;
#7939=EDGE_CURVE ( 'NONE', #27187, #37417, #17303, .T. ) ;
#7956=CARTESIAN_POINT ( 'NONE',  ( -5.177913976931298734, 78.94499979771843812, 5.372100000000002318 ) ) ;
#7958=CARTESIAN_POINT ( 'NONE',  ( -5.449044798931593547, 57.14999999999999858, 5.145813327217799049 ) ) ;
#7963=VECTOR ( 'NONE', #38861, 1000.000000000000000 ) ;
#7985=CARTESIAN_POINT ( 'NONE',  ( -14.39766717389552397, 60.02151067229126369, -1.904999999999999805 ) ) ;
#7986=ORIENTED_EDGE ( 'NONE', *, *, #41421, .F. ) ;
#7992=EDGE_CURVE ( 'NONE', #4862, #33118, #29487, .T. ) ;
#7997=CARTESIAN_POINT ( 'NONE',  ( -17.14499999999999957, 71.11999999999999034, -1.904999999999999583 ) ) ;
#8015=CARTESIAN_POINT ( 'NONE',  ( 5.571852488405371062, 78.91397923090406152, -5.086862008547680780 ) ) ;
#8022=VERTEX_POINT ( 'NONE', #21838 ) ;
#8024=ORIENTED_EDGE ( 'NONE', *, *, #2466, .F. ) ;
#8036=CARTESIAN_POINT ( 'NONE',  ( 13.34576682144454196, 17.14499999999997115, -5.016499999999998849 ) ) ;
#8045=DIRECTION ( 'NONE',  ( 0.9849462604886047856, 0.000000000000000000, 0.1728608224830407714 ) ) ;
#8047=DIRECTION ( 'NONE',  ( 0.000000000000000000, 1.000000000000000000, 0.000000000000000000 ) ) ;
#8076=AXIS2_PLACEMENT_3D ( 'NONE', #38255, #22657, #25468 ) ;
#8085=EDGE_LOOP ( 'NONE', ( #16010, #22347, #18581, #33928, #38964, #10390, #22184, #27259, #33297, #16982, #12121, #3599 ) ) ;
#8098=DIRECTION ( 'NONE',  ( 9.627370216492862708E-17, 1.000000000000000000, -0.000000000000000000 ) ) ;
#8100=CARTESIAN_POINT ( 'NONE',  ( -18.35410564743290607, 77.35382415001784295, 5.016499999999999737 ) ) ;
#8108=CARTESIAN_POINT ( 'NONE',  ( 17.14499999999999957, 71.11999999999999034, 5.016499999999999737 ) ) ;
#8111=DIRECTION ( 'NONE',  ( -1.000000000000000000, 1.365923996832131856E-16, 0.000000000000000000 ) ) ;
#8123=ORIENTED_EDGE ( 'NONE', *, *, #38619, .F. ) ;
#8128=DIRECTION ( 'NONE',  ( 9.627370216492862708E-17, 1.000000000000000000, -0.000000000000000000 ) ) ;
#8132=CIRCLE ( 'NONE', #31934, 6.349999999999999645 ) ;
#8134=CARTESIAN_POINT ( 'NONE',  ( 11.58677707360137532, 55.98894877578617724, 4.474811398758258285 ) ) ;
#8138=ORIENTED_EDGE ( 'NONE', *, *, #18745, .T. ) ;
#8155=CARTESIAN_POINT ( 'NONE',  ( -13.85159022459153988, 16.50999999999999801, -5.016499999999999737 ) ) ;
#8168=ADVANCED_FACE ( 'NONE', ( #9090, #42109 ), #32507, .F. ) ;
#8174=EDGE_CURVE ( 'NONE', #22720, #16450, #12904, .T. ) ;
#8179=ORIENTED_EDGE ( 'NONE', *, *, #15810, .T. ) ;
#8210=CARTESIAN_POINT ( 'NONE',  ( -20.83467972660109169, 65.95194780259438971, 5.016499999999999737 ) ) ;
#8224=CARTESIAN_POINT ( 'NONE',  ( 5.177913976931212581, 57.15000000000004832, -5.372100000000001430 ) ) ;
#8225=ADVANCED_FACE ( 'NONE', ( #6521 ), #25420, .F. ) ;
#8235=AXIS2_PLACEMENT_3D ( 'NONE', #32235, #35430, #38426 ) ;
#8239=AXIS2_PLACEMENT_3D ( 'NONE', #31929, #28096, #28726 ) ;
#8240=CARTESIAN_POINT ( 'NONE',  ( 13.17422243436029916, 17.14500000000093394, -5.016499999999999737 ) ) ;
#8249=CARTESIAN_POINT ( 'NONE',  ( 14.73199999999999754, 61.59499999999999886, -1.904999999999999583 ) ) ;
#8259=ORIENTED_EDGE ( 'NONE', *, *, #35338, .F. ) ;
#8261=ADVANCED_FACE ( 'NONE', ( #38901 ), #41473, .F. ) ;
#8267=CARTESIAN_POINT ( 'NONE',  ( 6.057513928997568797, 57.78500000000000369, -1.904999999999999805 ) ) ;
#8287=ORIENTED_EDGE ( 'NONE', *, *, #11633, .T. ) ;
#8292=ORIENTED_EDGE ( 'NONE', *, *, #42104, .T. ) ;
#8293=CIRCLE ( 'NONE', #31395, 2.540000000000000480 ) ;
#8295=AXIS2_PLACEMENT_3D ( 'NONE', #8680, #32262, #21644 ) ;
#8296=ORIENTED_EDGE ( 'NONE', *, *, #37593, .F. ) ;
#8308=CARTESIAN_POINT ( 'NONE',  ( 10.63219908769094069, 56.50600268266111215, 5.016499999999999737 ) ) ;
#8317=CARTESIAN_POINT ( 'NONE',  ( -11.25890006629606610, 56.90956307411701687, -5.016499999999999737 ) ) ;
#8337=ORIENTED_EDGE ( 'NONE', *, *, #2384, .T. ) ;
#8338=LINE ( 'NONE', #38781, #35787 ) ;
#8350=CARTESIAN_POINT ( 'NONE',  ( 11.58677707360137532, 55.24500000000000455, -4.474811398758259173 ) ) ;
#8366=CARTESIAN_POINT ( 'NONE',  ( -6.059261036834476144, 57.14999999999999858, -5.016499999999999737 ) ) ;
#8392=FACE_OUTER_BOUND ( 'NONE', #27755, .T. ) ;
#8411=EDGE_CURVE ( 'NONE', #18509, #33497, #35371, .T. ) ;
#8418=CARTESIAN_POINT ( 'NONE',  ( 6.057513928997551034, 86.35999999999998522, 1.904999999999996030 ) ) ;
#8475=CARTESIAN_POINT ( 'NONE',  ( 5.177913976931204587, 71.67999986514567468, 5.372100000000000541 ) ) ;
#8478=CARTESIAN_POINT ( 'NONE',  ( 14.73199999999999932, 12.96416000000000146, 0.000000000000000000 ) ) ;
#8486=CARTESIAN_POINT ( 'NONE',  ( -17.14499999999998892, 57.14999999999997726, -5.016499999999999737 ) ) ;
#8491=CARTESIAN_POINT ( 'NONE',  ( -11.41714695485569742, 57.14999999999998437, -5.016499999999999737 ) ) ;
#8509=ORIENTED_EDGE ( 'NONE', *, *, #24317, .F. ) ;
#8517=EDGE_CURVE ( 'NONE', #16752, #28439, #35646, .T. ) ;
#8520=CARTESIAN_POINT ( 'NONE',  ( -5.256666791691372076, 57.15000000000019043, -5.296388421271849722 ) ) ;
#8522=CARTESIAN_POINT ( 'NONE',  ( 10.94257363143051087, 56.35470871607771670, 4.428493390990901446 ) ) ;
#8523=CARTESIAN_POINT ( 'NONE',  ( -6.059261036834472591, 56.98375738874752727, -5.016500000000000625 ) ) ;
#8532=CARTESIAN_POINT ( 'NONE',  ( -11.58677707360117282, 55.41127257906206438, -4.474811398756911807 ) ) ;
#8541=CIRCLE ( 'NONE', #33701, 12.69999999999999751 ) ;
#8552=ORIENTED_EDGE ( 'NONE', *, *, #35525, .F. ) ;
#8555=SURFACE_STYLE_FILL_AREA ( #14714 ) ;
#8582=DIRECTION ( 'NONE',  ( 1.000000000000000000, 0.000000000000000000, 0.000000000000000000 ) ) ;
#8583=CARTESIAN_POINT ( 'NONE',  ( -5.486567272856878414E-14, 86.35999999999998522, 0.000000000000000000 ) ) ;
#8584=CARTESIAN_POINT ( 'NONE',  ( 7.213960532363571154, 78.77618639008812806, -1.904999999999999583 ) ) ;
#8587=ORIENTED_EDGE ( 'NONE', *, *, #32686, .T. ) ;
#8622=CARTESIAN_POINT ( 'NONE',  ( 17.68910244842765778, 8.844871939465424049, 0.000000000000000000 ) ) ;
#8626=CARTESIAN_POINT ( 'NONE',  ( -5.871452009091383317, 65.30181249999998272, -5.016499999999999737 ) ) ;
#8629=B_SPLINE_CURVE_WITH_KNOTS ( 'NONE', 5,
 ( #30360, #20972, #23750, #14369, #39978, #36770, #583, #20549 ),
 .UNSPECIFIED., .F., .F.,
 ( 6, 2, 6 ),
 ( -5.999999999695239656E-08, 0.0004919218780628863792, 0.0009839037561257695831 ),
 .UNSPECIFIED. ) ;
#8649=CARTESIAN_POINT ( 'NONE',  ( -5.579075174912628832, 56.51499999999997925, -4.418274828058819992 ) ) ;
#8675=PLANE ( 'NONE',  #4977 ) ;
#8680=CARTESIAN_POINT ( 'NONE',  ( 1.204770341778093456E-15, 12.51401280605345967, 0.000000000000000000 ) ) ;
#8700=LINE ( 'NONE', #28289, #32035 ) ;
#8708=PRODUCT_DEFINITION_FORMATION_WITH_SPECIFIED_SOURCE ( 'ANY', '', #30001, .NOT_KNOWN. ) ;
#8720=EDGE_CURVE ( 'NONE', #20977, #16752, #40821, .T. ) ;
#8721=ORIENTED_EDGE ( 'NONE', *, *, #16216, .F. ) ;
#8724=CARTESIAN_POINT ( 'NONE',  ( 17.68910244842765778, -7.669212195657745698E-17, 0.000000000000000000 ) ) ;
#8727=CARTESIAN_POINT ( 'NONE',  ( -14.73199999999999399, 17.14499999999999957, 0.000000000000000000 ) ) ;
#8734=EDGE_CURVE ( 'NONE', #25703, #39961, #29523, .T. ) ;
#8736=VERTEX_POINT ( 'NONE', #25173 ) ;
#8754=ORIENTED_EDGE ( 'NONE', *, *, #13430, .F. ) ;
#8758=VECTOR ( 'NONE', #35203, 1000.000000000000000 ) ;
#8764=ORIENTED_EDGE ( 'NONE', *, *, #41268, .F. ) ;
#8769=DIRECTION ( 'NONE',  ( -1.000000000000000000, 0.000000000000000000, 0.000000000000000000 ) ) ;
#8778=ORIENTED_EDGE ( 'NONE', *, *, #9517, .F. ) ;
#8783=CARTESIAN_POINT ( 'NONE',  ( 6.113380087472956159E-17, 0.6350000000000001199, 0.000000000000000000 ) ) ;
#8800=CYLINDRICAL_SURFACE ( 'NONE', #16099, 2.540000000000000480 ) ;
#8803=ORIENTED_EDGE ( 'NONE', *, *, #27463, .T. ) ;
#8841=CARTESIAN_POINT ( 'NONE',  ( -5.241362157049125337, 65.30181249999998272, -5.310945289804168468 ) ) ;
#8844=EDGE_LOOP ( 'NONE', ( #26773, #19969, #18010, #36197, #36479 ) ) ;
#8847=DIRECTION ( 'NONE',  ( 9.627370216492862708E-17, 1.000000000000000000, -0.000000000000000000 ) ) ;
#8853=CARTESIAN_POINT ( 'NONE',  ( 5.421568387540328438, 78.92574702321223867, -5.165409981420356011 ) ) ;
#8862=ORIENTED_EDGE ( 'NONE', *, *, #39176, .T. ) ;
#8864=CARTESIAN_POINT ( 'NONE',  ( 10.92199999999999704, 17.14499999999999957, 5.850485014536587995E-17 ) ) ;
#8877=ORIENTED_EDGE ( 'NONE', *, *, #19024, .T. ) ;
#8880=DIRECTION ( 'NONE',  ( -1.000000000000000000, 1.365923996832131856E-16, 0.000000000000000000 ) ) ;
#8886=CARTESIAN_POINT ( 'NONE',  ( 5.256643466843669010, 57.15000000000020464, -5.296410794270209443 ) ) ;
#8889=VECTOR ( 'NONE', #34605, 1000.000000000000000 ) ;
#8893=ORIENTED_EDGE ( 'NONE', *, *, #33827, .T. ) ;
#8901=ADVANCED_FACE ( 'NONE', ( #2189 ), #9198, .F. ) ;
#8902=ORIENTED_EDGE ( 'NONE', *, *, #2707, .T. ) ;
#8904=CARTESIAN_POINT ( 'NONE',  ( -7.213960532363670630, 78.77618639008812806, 1.904999999999999583 ) ) ;
#8932=EDGE_CURVE ( 'NONE', #17444, #1544, #41157, .T. ) ;
#8936=CARTESIAN_POINT ( 'NONE',  ( -5.224239234539626686, 57.14999999999513136, -5.327449267724884585 ) ) ;
#8946=CARTESIAN_POINT ( 'NONE',  ( -17.14499999999999957, 71.11999999999999034, 5.016499999999999737 ) ) ;
#8972=ORIENTED_EDGE ( 'NONE', *, *, #27922, .F. ) ;
#8980=CARTESIAN_POINT ( 'NONE',  ( 12.21488373879589417, 55.24500000000000455, -5.016499999999999737 ) ) ;
#8993=DIRECTION ( 'NONE',  ( 6.353134868986659519E-16, -1.000000000000000000, 0.000000000000000000 ) ) ;
#8998=ADVANCED_FACE ( 'NONE', ( #33981 ), #32634, .F. ) ;
#9010=CARTESIAN_POINT ( 'NONE',  ( -17.14499999999999957, 71.11999999999999034, 5.016499999999999737 ) ) ;
#9026=ORIENTED_EDGE ( 'NONE', *, *, #14841, .F. ) ;
#9028=CARTESIAN_POINT ( 'NONE',  ( 13.85159022459153988, 12.96416000000000146, -5.016499999999999737 ) ) ;
#9056=CARTESIAN_POINT ( 'NONE',  ( 6.113380087472956159E-17, 0.6350000000000001199, 0.000000000000000000 ) ) ;
#9068=CARTESIAN_POINT ( 'NONE',  ( 4.792324638223571576, 56.51998046905274009, -4.972049999999996750 ) ) ;
#9090=FACE_BOUND ( 'NONE', #33686, .T. ) ;
#9094=ORIENTED_EDGE ( 'NONE', *, *, #39789, .T. ) ;
#9103=CARTESIAN_POINT ( 'NONE',  ( 4.825814575782076510, 56.51499999999999346, -4.829586058641568869 ) ) ;
#9107=CARTESIAN_POINT ( 'NONE',  ( -5.570375128628924699, 56.51499999999999346, 4.419987129958256489 ) ) ;
#9128=CARTESIAN_POINT ( 'NONE',  ( -14.80692295515835255, 78.04183178746349370, 5.016499999999999737 ) ) ;
#9156=CARTESIAN_POINT ( 'NONE',  ( -6.059261036834474368, 56.51499999999998636, -4.381499999999999950 ) ) ;
#9168=LINE ( 'NONE', #22124, #19660 ) ;
#9185=LINE ( 'NONE', #34749, #37843 ) ;
#9198=PLANE ( 'NONE',  #30594 ) ;
#9200=CARTESIAN_POINT ( 'NONE',  ( -13.76130258807007678, 16.83823567964706314, 5.016499999999998849 ) ) ;
#9203=CARTESIAN_POINT ( 'NONE',  ( -17.14499999999999957, 71.11999999999999034, 5.016499999999999737 ) ) ;
#9209=EDGE_CURVE ( 'NONE', #38242, #32125, #25582, .T. ) ;
#9219=CYLINDRICAL_SURFACE ( 'NONE', #23944, 6.349999999999999645 ) ;
#9224=EDGE_CURVE ( 'NONE', #1883, #37954, #10180, .T. ) ;
#9225=CARTESIAN_POINT ( 'NONE',  ( 5.664977208693820820, 53.58606249999999704, 5.033228321271210781 ) ) ;
#9251=DIRECTION ( 'NONE',  ( 6.353134868986659519E-16, -1.000000000000000000, 0.000000000000000000 ) ) ;
#9265=CARTESIAN_POINT ( 'NONE',  ( -5.305748947172281405, 65.30181249999998272, -5.247078976224250013 ) ) ;
#9267=ADVANCED_FACE ( 'NONE', ( #13438 ), #38, .F. ) ;
#9274=ORIENTED_EDGE ( 'NONE', *, *, #877, .F. ) ;
#9319=CARTESIAN_POINT ( 'NONE',  ( 6.059261036834404202, 56.58343591620776181, -4.712961528314684401 ) ) ;
#9341=CIRCLE ( 'NONE', #34526, 7.461249999999999716 ) ;
#9347=CYLINDRICAL_SURFACE ( 'NONE', #30704, 0.6350000000000001199 ) ;
#9359=ORIENTED_EDGE ( 'NONE', *, *, #392, .T. ) ;
#9365=DIRECTION ( 'NONE',  ( 6.353134868986659519E-16, -1.000000000000000000, 0.000000000000000000 ) ) ;
#9372=DIRECTION ( 'NONE',  ( -0.9891443546370349837, 0.000000000000000000, -0.1469470846586743706 ) ) ;
#9377=EDGE_LOOP ( 'NONE', ( #16271, #25100, #2920, #22073 ) ) ;
#9384=ORIENTED_EDGE ( 'NONE', *, *, #18506, .T. ) ;
#9387=( NAMED_UNIT ( * ) SI_UNIT ( $, .STERADIAN. ) SOLID_ANGLE_UNIT ( ) );
#9389=CARTESIAN_POINT ( 'NONE',  ( -14.95453923199683288, 61.75387968257833649, -5.016499999999999737 ) ) ;
#9396=ORIENTED_EDGE ( 'NONE', *, *, #9706, .T. ) ;
#9416=DIRECTION ( 'NONE',  ( -1.000000000000000000, 0.000000000000000000, 0.000000000000000000 ) ) ;
#9422=CARTESIAN_POINT ( 'NONE',  ( 5.241362157049035631, 77.01756249999996840, 5.310945289804168468 ) ) ;
#9423=ORIENTED_EDGE ( 'NONE', *, *, #586, .F. ) ;
#9453=CARTESIAN_POINT ( 'NONE',  ( -14.39766717389550443, 30.83083951148099189, -1.904999999999999805 ) ) ;
#9457=EDGE_CURVE ( 'NONE', #3896, #31942, #24, .T. ) ;
#9459=CIRCLE ( 'NONE', #29193, 2.540000000000000480 ) ;
#9485=FACE_OUTER_BOUND ( 'NONE', #41835, .T. ) ;
#9517=EDGE_CURVE ( 'NONE', #4652, #449, #14772, .T. ) ;
#9545=ORIENTED_EDGE ( 'NONE', *, *, #19123, .T. ) ;
#9548=DIRECTION ( 'NONE',  ( 0.000000000000000000, 0.000000000000000000, -1.000000000000000000 ) ) ;
#9553=PLANE ( 'NONE',  #17199 ) ;
#9569=VECTOR ( 'NONE', #28982, 1000.000000000000000 ) ;
#9589=ORIENTED_EDGE ( 'NONE', *, *, #32177, .T. ) ;
#9605=CIRCLE ( 'NONE', #33428, 2.540000000000000480 ) ;
#9606=CARTESIAN_POINT ( 'NONE',  ( 10.39494437172059094, 56.51500000000000057, 5.094799277214218769 ) ) ;
#9609=LINE ( 'NONE', #22577, #879 ) ;
#9633=VERTEX_POINT ( 'NONE', #5754 ) ;
#9655=EDGE_CURVE ( 'NONE', #10059, #1007, #15209, .T. ) ;
#9661=CARTESIAN_POINT ( 'NONE',  ( 6.349999999999963229, 57.14999999999999858, 0.000000000000000000 ) ) ;
#9665=CARTESIAN_POINT ( 'NONE',  ( -11.66725022231030628, 17.14499999999999957, 5.016499999999999737 ) ) ;
#9670=LINE ( 'NONE', #35671, #22014 ) ;
#9673=CARTESIAN_POINT ( 'NONE',  ( -5.305748947172302721, 88.73331249999998249, 5.247078976224250013 ) ) ;
#9682=ORIENTED_EDGE ( 'NONE', *, *, #19865, .T. ) ;
#9706=EDGE_CURVE ( 'NONE', #5873, #17114, #14282, .T. ) ;
#9717=DIRECTION ( 'NONE',  ( 0.000000000000000000, 1.000000000000000000, 0.000000000000000000 ) ) ;
#9724=CARTESIAN_POINT ( 'NONE',  ( -10.28897677580358305, 57.14999999999998437, -4.381499999999999950 ) ) ;
#9725=CARTESIAN_POINT ( 'NONE',  ( -19.68500000000000227, 71.11999999999999034, 5.016499999999999737 ) ) ;
#9746=CARTESIAN_POINT ( 'NONE',  ( 5.322370864742547170, 56.51500000000019952, 5.239063871132564998 ) ) ;
#9751=ORIENTED_EDGE ( 'NONE', *, *, #6848, .T. ) ;
#9756=DIRECTION ( 'NONE',  ( -0.000000000000000000, -0.000000000000000000, -1.000000000000000000 ) ) ;
#9757=TOROIDAL_SURFACE ( 'NONE', #31522, 14.09699999999999420, 0.6350000000000000089 ) ;
#9759=ORIENTED_EDGE ( 'NONE', *, *, #18596, .T. ) ;
#9761=FACE_OUTER_BOUND ( 'NONE', #8844, .T. ) ;
#9765=CARTESIAN_POINT ( 'NONE',  ( -5.941785710907115714, 57.15000000000771507, -5.016499999999997961 ) ) ;
#9773=CARTESIAN_POINT ( 'NONE',  ( 5.177913976931196594, 78.94499979771845233, 5.372100000000001430 ) ) ;
#9775=FACE_OUTER_BOUND ( 'NONE', #15304, .T. ) ;
#9787=CARTESIAN_POINT ( 'NONE',  ( 5.578816284158309990, 56.51499999999997215, -4.418322536902425490 ) ) ;
#9808=AXIS2_PLACEMENT_3D ( 'NONE', #13444, #26004, #6427 ) ;
#9811=ADVANCED_FACE ( 'NONE', ( #32134 ), #22309, .T. ) ;
#9817=CARTESIAN_POINT ( 'NONE',  ( -14.95453923199683643, 61.75387968257833649, 5.016499999999999737 ) ) ;
#9819=CARTESIAN_POINT ( 'NONE',  ( 1.650612623617701257E-15, 17.14499999999999957, 0.000000000000000000 ) ) ;
#9840=CARTESIAN_POINT ( 'NONE',  ( 5.177913976931193041, 88.73331249999999670, 5.372100000000000541 ) ) ;
#9849=CARTESIAN_POINT ( 'NONE',  ( -11.66725022231030984, 17.14499999999999957, -5.016499999999999737 ) ) ;
#9864=VECTOR ( 'NONE', #28268, 1000.000000000000000 ) ;
#9877=CARTESIAN_POINT ( 'NONE',  ( -5.664977208693910526, 77.01756250000002524, 5.033228321271210781 ) ) ;
#9891=CARTESIAN_POINT ( 'NONE',  ( 5.892673590944617956, 78.88814725119658533, -5.017439957471150791 ) ) ;
#9899=ORIENTED_EDGE ( 'NONE', *, *, #23307, .T. ) ;
#9910=ADVANCED_FACE ( 'NONE', ( #9761 ), #2440, .F. ) ;
#9915=ORIENTED_EDGE ( 'NONE', *, *, #12125, .F. ) ;
#9933=EDGE_CURVE ( 'NONE', #13136, #18529, #37646, .T. ) ;
#9950=CARTESIAN_POINT ( 'NONE',  ( -7.213960532363674183, 86.35999999999998522, -1.904999999999999805 ) ) ;
#9958=VECTOR ( 'NONE', #26969, 1000.000000000000227 ) ;
#9970=CARTESIAN_POINT ( 'NONE',  ( -6.059261036834476144, 56.51499999999998636, -5.016499999999990855 ) ) ;
#9971=AXIS2_PLACEMENT_3D ( 'NONE', #19541, #3169, #41944 ) ;
#10023=CARTESIAN_POINT ( 'NONE',  ( -12.69999999999999574, 16.51000000000000156, 0.000000000000000000 ) ) ;
#10026=LINE ( 'NONE', #10449, #16344 ) ;
#10027=EDGE_CURVE ( 'NONE', #700, #16922, #31850, .T. ) ;
#10032=DIRECTION ( 'NONE',  ( -1.000000000000000000, -1.092739197465705287E-15, 0.000000000000000000 ) ) ;
#10039=CARTESIAN_POINT ( 'NONE',  ( 20.83467972660109169, 65.95194780259438971, 5.016499999999999737 ) ) ;
#10043=LINE ( 'NONE', #42021, #40946 ) ;
#10052=ORIENTED_EDGE ( 'NONE', *, *, #27169, .F. ) ;
#10059=VERTEX_POINT ( 'NONE', #23578 ) ;
#10075=AXIS2_PLACEMENT_3D ( 'NONE', #3382, #16349, #25530 ) ;
#10089=CARTESIAN_POINT ( 'NONE',  ( -6.059261036834497460, 88.73331249999998249, 5.016499999999999737 ) ) ;
#10109=CARTESIAN_POINT ( 'NONE',  ( -17.14499999999999957, 71.11999999999999034, 1.904999999999989146 ) ) ;
#10140=B_SPLINE_CURVE_WITH_KNOTS ( 'NONE', 3,
 ( #5072, #34240, #18023, #15252, #28039, #41048 ),
 .UNSPECIFIED., .F., .F.,
 ( 4, 2, 4 ),
 ( -0.0001503376881350242306, 0.0002168025613753844804, 0.0005839428108857932457 ),
 .UNSPECIFIED. ) ;
#10155=CARTESIAN_POINT ( 'NONE',  ( 16.87828382557106721, 17.14499999999999957, 0.000000000000000000 ) ) ;
#10169=ORIENTED_EDGE ( 'NONE', *, *, #33432, .T. ) ;
#10176=CARTESIAN_POINT ( 'NONE',  ( 5.177913976931215245, 56.99702125087947024, 5.372099999999998765 ) ) ;
#10180=CIRCLE ( 'NONE', #34016, 0.6350000000000001199 ) ;
#10183=CARTESIAN_POINT ( 'NONE',  ( -5.860279866612252420, 56.51500000000000057, -5.019549989587524408 ) ) ;
#10186=FACE_OUTER_BOUND ( 'NONE', #25932, .T. ) ;
#10191=CARTESIAN_POINT ( 'NONE',  ( -5.506767014370270275, 78.91949168437545836, -5.113098386149694363 ) ) ;
#10198=DIRECTION ( 'NONE',  ( 0.9891443546370349837, 0.000000000000000000, 0.1469470846586742874 ) ) ;
#10233=DIRECTION ( 'NONE',  ( -0.000000000000000000, -0.000000000000000000, -1.000000000000000000 ) ) ;
#10234=EDGE_CURVE ( 'NONE', #20064, #8022, #17196, .T. ) ;
#10240=DIRECTION ( 'NONE',  ( -9.627370216492862708E-17, -1.000000000000000000, 0.000000000000000000 ) ) ;
#10248=CARTESIAN_POINT ( 'NONE',  ( -10.28897677580358128, 57.14999999999998437, -5.016499999999999737 ) ) ;
#10256=DIRECTION ( 'NONE',  ( 0.1715592850456333085, -0.1224830539174543292, 0.9775302108976914317 ) ) ;
#10259=VERTEX_POINT ( 'NONE', #1250 ) ;
#10273=CARTESIAN_POINT ( 'NONE',  ( -5.486567272856878414E-14, 86.35999999999998522, 0.000000000000000000 ) ) ;
#10285=ADVANCED_FACE ( 'NONE', ( #11225, #4026 ), #4654, .F. ) ;
#10287=ADVANCED_FACE ( 'NONE', ( #1454 ), #40840, .T. ) ;
#10300=VECTOR ( 'NONE', #13334, 1000.000000000000000 ) ;
#10304=CARTESIAN_POINT ( 'NONE',  ( -5.475330206976889436, 77.01756250000002524, 5.107412922131463695 ) ) ;
#10305=CARTESIAN_POINT ( 'NONE',  ( -5.813441077435913762, 56.51499999999999346, 4.384678760708306200 ) ) ;
#10325=CARTESIAN_POINT ( 'NONE',  ( 5.871452009091314039, 57.14999999999999858, -5.016499999999999737 ) ) ;
#10367=DIRECTION ( 'NONE',  ( -6.353134868986659519E-16, 1.000000000000000000, 0.000000000000000000 ) ) ;
#10372=PLANE ( 'NONE',  #1769 ) ;
#10373=AXIS2_PLACEMENT_3D ( 'NONE', #6018, #8993, #25588 ) ;
#10390=ORIENTED_EDGE ( 'NONE', *, *, #6379, .T. ) ;
#10392=DIRECTION ( 'NONE',  ( -0.1469470846586743706, -9.335746474409589170E-17, -0.9891443546370348727 ) ) ;
#10402=DIRECTION ( 'NONE',  ( -0.1715592850456333363, 0.1224830539174543431, 0.9775302108976914317 ) ) ;
#10441=EDGE_CURVE ( 'NONE', #1883, #11997, #34036, .T. ) ;
#10448=AXIS2_PLACEMENT_3D ( 'NONE', #28013, #2480, #28230 ) ;
#10449=CARTESIAN_POINT ( 'NONE',  ( -3.745035802202505265E-14, 57.78499999999999659, -1.904999999999999805 ) ) ;
#10453=AXIS2_PLACEMENT_3D ( 'NONE', #5964, #34932, #18923 ) ;
#10463=CARTESIAN_POINT ( 'NONE',  ( -5.800481910058950419, 78.89561208401060810, 5.028344476440693711 ) ) ;
#10475=ORIENTED_EDGE ( 'NONE', *, *, #5011, .F. ) ;
#10482=EDGE_LOOP ( 'NONE', ( #23465, #21341, #19368, #8292 ) ) ;
#10514=CARTESIAN_POINT ( 'NONE',  ( -6.059261036834474368, 53.58606250000000415, 5.016499999999999737 ) ) ;
#10523=ORIENTED_EDGE ( 'NONE', *, *, #41005, .T. ) ;
#10535=CARTESIAN_POINT ( 'NONE',  ( 6.059261036834394432, 71.63300248836196715, 5.016499999999999737 ) ) ;
#10537=ORIENTED_EDGE ( 'NONE', *, *, #40728, .F. ) ;
#10567=AXIS2_PLACEMENT_3D ( 'NONE', #2997, #41971, #9372 ) ;
#10597=ORIENTED_EDGE ( 'NONE', *, *, #6446, .T. ) ;
#10600=DIRECTION ( 'NONE',  ( 6.353134868986659519E-16, -1.000000000000000000, 0.000000000000000000 ) ) ;
#10628=AXIS2_PLACEMENT_3D ( 'NONE', #37178, #41004, #11810 ) ;
#10661=FACE_OUTER_BOUND ( 'NONE', #36667, .T. ) ;
#10668=LINE ( 'NONE', #4097, #34745 ) ;
#10671=AXIS2_PLACEMENT_3D ( 'NONE', #28360, #14932, #25167 ) ;
#10673=CARTESIAN_POINT ( 'NONE',  ( -5.451267667241070720E-14, 85.80437499999999318, 0.000000000000000000 ) ) ;
#10678=CYLINDRICAL_SURFACE ( 'NONE', #40105, 2.539999999999999591 ) ;
#10696=ORIENTED_EDGE ( 'NONE', *, *, #39789, .F. ) ;
#10719=FACE_OUTER_BOUND ( 'NONE', #33667, .T. ) ;
#10727=ORIENTED_EDGE ( 'NONE', *, *, #19352, .F. ) ;
#10762=DIRECTION ( 'NONE',  ( -5.463695987328526437E-16, -1.000000000000000000, -1.672774450599033775E-31 ) ) ;
#10766=EDGE_CURVE ( 'NONE', #6407, #1559, #18144, .T. ) ;
#10789=CYLINDRICAL_SURFACE ( 'NONE', #17666, 1.270000000000000240 ) ;
#10795=CARTESIAN_POINT ( 'NONE',  ( 5.941785710906973605, 57.15000000000325997, 5.016500000000000625 ) ) ;
#10799=ORIENTED_EDGE ( 'NONE', *, *, #28499, .F. ) ;
#10804=CIRCLE ( 'NONE', #11465, 6.349999999999999645 ) ;
#10828=TOROIDAL_SURFACE ( 'NONE', #42142, 15.36699999999999555, 0.6350000000000000089 ) ;
#10865=DIRECTION ( 'NONE',  ( 1.000000000000000000, -9.627370216492862708E-17, 0.000000000000000000 ) ) ;
#10871=CARTESIAN_POINT ( 'NONE',  ( 12.21488373879589062, 55.24500000000000455, 5.016499999999999737 ) ) ;
#10879=CARTESIAN_POINT ( 'NONE',  ( -5.974493989214139766, 78.88147413144915276, 5.016500000000001513 ) ) ;
#10880=FACE_OUTER_BOUND ( 'NONE', #30927, .T. ) ;
#10883=DIRECTION ( 'NONE',  ( 1.000000000000000000, 0.000000000000000000, 0.000000000000000000 ) ) ;
#10889=CARTESIAN_POINT ( 'NONE',  ( -3.630816577625875226E-14, 57.14999999999999147, 0.000000000000000000 ) ) ;
#10895=ORIENTED_EDGE ( 'NONE', *, *, #6446, .F. ) ;
#10909=CARTESIAN_POINT ( 'NONE',  ( 11.62920297224776611, 55.59919541885983563, -5.016499999999893156 ) ) ;
#10911=EDGE_CURVE ( 'NONE', #30952, #1883, #16309, .T. ) ;
#10923=CARTESIAN_POINT ( 'NONE',  ( 10.92199999999999704, 57.78500000000000369, 5.016499999999999737 ) ) ;
#10926=AXIS2_PLACEMENT_3D ( 'NONE', #36123, #16503, #13102 ) ;
#10928=CARTESIAN_POINT ( 'NONE',  ( -4.737240446979679831, 56.51499999999999346, 4.914900000000012703 ) ) ;
#10935=DIRECTION ( 'NONE',  ( -0.000000000000000000, -1.000000000000000000, -0.000000000000000000 ) ) ;
#10948=VERTEX_POINT ( 'NONE', #38697 ) ;
#10964=DIRECTION ( 'NONE',  ( -6.353134868986659519E-16, 1.000000000000000000, 0.000000000000000000 ) ) ;
#10998=ORIENTED_EDGE ( 'NONE', *, *, #25402, .T. ) ;
#11003=CARTESIAN_POINT ( 'NONE',  ( 13.51778232847667205, 17.08230797367789222, 5.016499999999999737 ) ) ;
#11013=EDGE_CURVE ( 'NONE', #19376, #449, #4091, .T. ) ;
#11027=DIRECTION ( 'NONE',  ( -9.627370216492862708E-17, -1.000000000000000000, 0.000000000000000000 ) ) ;
#11050=CARTESIAN_POINT ( 'NONE',  ( 12.21488373879589240, 55.24500000000000455, 5.016499999999999737 ) ) ;
#11069=VERTEX_POINT ( 'NONE', #13959 ) ;
#11074=CIRCLE ( 'NONE', #24642, 6.350000000000004974 ) ;
#11077=CARTESIAN_POINT ( 'NONE',  ( -5.871452009091383317, 57.14999999999999147, 5.016499999999999737 ) ) ;
#11082=AXIS2_PLACEMENT_3D ( 'NONE', #26401, #32375, #29389 ) ;
#11108=ORIENTED_EDGE ( 'NONE', *, *, #36604, .T. ) ;
#11109=ORIENTED_EDGE ( 'NONE', *, *, #8932, .T. ) ;
#11123=CARTESIAN_POINT ( 'NONE',  ( 12.21488373878702305, 55.49440886859300548, -5.016500000000000625 ) ) ;
#11124=AXIS2_PLACEMENT_3D ( 'NONE', #30211, #17835, #5089 ) ;
#11132=CARTESIAN_POINT ( 'NONE',  ( -11.55299880265467394, 55.57741982016696625, 4.472382752598255351 ) ) ;
#11135=CARTESIAN_POINT ( 'NONE',  ( 16.62722885652246418, 62.94807988814252298, 4.514343177587269551 ) ) ;
#11160=ORIENTED_EDGE ( 'NONE', *, *, #24839, .F. ) ;
#11174=CARTESIAN_POINT ( 'NONE',  ( 10.92199999999999704, 56.51500000000000057, 5.016499999999999737 ) ) ;
#11186=B_SPLINE_CURVE_WITH_KNOTS ( 'NONE', 3,
 ( #3770, #29734, #20541, #40382, #14159, #23954 ),
 .UNSPECIFIED., .F., .F.,
 ( 4, 2, 4 ),
 ( 0.000000000000000000, 0.4601069123251853576, 0.9202138246503707153 ),
 .UNSPECIFIED. ) ;
#11189=VERTEX_POINT ( 'NONE', #13757 ) ;
#11193=ORIENTED_EDGE ( 'NONE', *, *, #11494, .T. ) ;
#11201=EDGE_CURVE ( 'NONE', #32125, #1397, #29043, .T. ) ;
#11204=EDGE_CURVE ( 'NONE', #31590, #3167, #40177, .T. ) ;
#11222=FACE_OUTER_BOUND ( 'NONE', #815, .T. ) ;
#11223=ORIENTED_EDGE ( 'NONE', *, *, #4045, .F. ) ;
#11225=FACE_OUTER_BOUND ( 'NONE', #11985, .T. ) ;
#11231=CARTESIAN_POINT ( 'NONE',  ( 13.85159022459153988, 12.96416000000000146, -5.016499999999999737 ) ) ;
#11234=CARTESIAN_POINT ( 'NONE',  ( 13.85159022459153988, 12.96416000000000146, -5.016499999999999737 ) ) ;
#11239=CARTESIAN_POINT ( 'NONE',  ( -10.28897677580358305, 57.14999999999998437, 5.016499999999999737 ) ) ;
#11250=EDGE_CURVE ( 'NONE', #35053, #3380, #17487, .T. ) ;
#11260=CARTESIAN_POINT ( 'NONE',  ( 6.059261036834384662, 77.01756249999996840, -5.016499999999999737 ) ) ;
#11275=ORIENTED_EDGE ( 'NONE', *, *, #23821, .F. ) ;
#11280=EDGE_LOOP ( 'NONE', ( #36640, #19553, #17378, #21240 ) ) ;
#11288=CARTESIAN_POINT ( 'NONE',  ( 14.80692295515832058, 78.04183178746352212, -5.016499999999999737 ) ) ;
#11294=VECTOR ( 'NONE', #5440, 1000.000000000000000 ) ;
#11300=CARTESIAN_POINT ( 'NONE',  ( -11.11710224467015351, 56.30409367656761788, -5.016499999999996184 ) ) ;
#11303=DIRECTION ( 'NONE',  ( -0.000000000000000000, 1.000000000000000000, -0.000000000000000000 ) ) ;
#11319=CARTESIAN_POINT ( 'NONE',  ( 17.68910244842765778, 0.6349999999999984546, 0.000000000000000000 ) ) ;
#11332=FACE_OUTER_BOUND ( 'NONE', #37421, .T. ) ;
#11342=CARTESIAN_POINT ( 'NONE',  ( -10.62867326514792410, 56.48194529650098872, 4.405924061720235763 ) ) ;
#11347=CARTESIAN_POINT ( 'NONE',  ( 1.650612623617701257E-15, 17.14499999999999957, 0.000000000000000000 ) ) ;
#11357=EDGE_LOOP ( 'NONE', ( #12775, #34408, #17188, #20825 ) ) ;
#11384=DIRECTION ( 'NONE',  ( -0.000000000000000000, -0.000000000000000000, -1.000000000000000000 ) ) ;
#11393=DIRECTION ( 'NONE',  ( 6.353134868986659519E-16, -1.000000000000000000, 0.000000000000000000 ) ) ;
#11401=ORIENTED_EDGE ( 'NONE', *, *, #39176, .F. ) ;
#11406=CARTESIAN_POINT ( 'NONE',  ( 5.692269266617126178, 78.90431106374074943, -5.047924920909481195 ) ) ;
#11444=VERTEX_POINT ( 'NONE', #37791 ) ;
#11447=DIRECTION ( 'NONE',  ( 1.000000000000000000, 0.000000000000000000, 0.000000000000000000 ) ) ;
#11450=CARTESIAN_POINT ( 'NONE',  ( -6.059261036834475256, 57.15000000000000568, 5.016499999999999737 ) ) ;
#11451=ORIENTED_EDGE ( 'NONE', *, *, #3434, .F. ) ;
#11461=CARTESIAN_POINT ( 'NONE',  ( 5.241362157049035631, 88.73331249999999670, -5.310945289804168468 ) ) ;
#11465=AXIS2_PLACEMENT_3D ( 'NONE', #30465, #23004, #10032 ) ;
#11469=ORIENTED_EDGE ( 'NONE', *, *, #11519, .F. ) ;
#11484=SHAPE_REPRESENTATION ( 'Corkscrew Body', ( #3275 ), #40037 ) ;
#11485=DIRECTION ( 'NONE',  ( -1.000000000000000000, 0.000000000000000000, 0.000000000000000000 ) ) ;
#11492=CARTESIAN_POINT ( 'NONE',  ( 10.96186877710231755, 56.39406130473820156, 5.016499999999998849 ) ) ;
#11493=DIRECTION ( 'NONE',  ( -1.000000000000000000, 0.000000000000000000, 0.000000000000000000 ) ) ;
#11494=EDGE_CURVE ( 'NONE', #38361, #21382, #11074, .T. ) ;
#11496=ORIENTED_EDGE ( 'NONE', *, *, #40277, .T. ) ;
#11502=CARTESIAN_POINT ( 'NONE',  ( 17.14499999999999957, 71.11999999999999034, -1.904999999999999583 ) ) ;
#11513=ORIENTED_EDGE ( 'NONE', *, *, #406, .F. ) ;
#11519=EDGE_CURVE ( 'NONE', #22696, #31590, #4815, .T. ) ;
#11536=ORIENTED_EDGE ( 'NONE', *, *, #39798, .F. ) ;
#11558=CARTESIAN_POINT ( 'NONE',  ( -11.66725022231030984, 55.24499999999999034, 5.016499999999999737 ) ) ;
#11564=ORIENTED_EDGE ( 'NONE', *, *, #34197, .F. ) ;
#11585=VERTEX_POINT ( 'NONE', #12015 ) ;
#11599=ORIENTED_EDGE ( 'NONE', *, *, #37833, .T. ) ;
#11602=CARTESIAN_POINT ( 'NONE',  ( -14.73199999999999932, 12.96416000000000146, 0.000000000000000000 ) ) ;
#11623=ORIENTED_EDGE ( 'NONE', *, *, #32030, .F. ) ;
#11633=EDGE_CURVE ( 'NONE', #34925, #11585, #22211, .T. ) ;
#11639=AXIS2_PLACEMENT_3D ( 'NONE', #31982, #31559, #11752 ) ;
#11643=VERTEX_POINT ( 'NONE', #12855 ) ;
#11652=CARTESIAN_POINT ( 'NONE',  ( 5.511275327887530828, 56.51500000000046242, -5.111309966001113203 ) ) ;
#11655=VECTOR ( 'NONE', #14716, 1000.000000000000114 ) ;
#11659=VERTEX_POINT ( 'NONE', #41640 ) ;
#11662=VECTOR ( 'NONE', #16522, 1000.000000000000000 ) ;
#11703=AXIS2_PLACEMENT_3D ( 'NONE', #5192, #27952, #2204 ) ;
#11704=FACE_OUTER_BOUND ( 'NONE', #31053, .T. ) ;
#11707=CARTESIAN_POINT ( 'NONE',  ( -6.059261036834472591, 56.51499999999997925, -4.547742611252458822 ) ) ;
#11709=EDGE_LOOP ( 'NONE', ( #5989, #3292, #22617, #23328 ) ) ;
#11710=VERTEX_POINT ( 'NONE', #9661 ) ;
#11724=CARTESIAN_POINT ( 'NONE',  ( 17.14499999999999957, 71.11999999999999034, 5.016499999999999737 ) ) ;
#11728=ORIENTED_EDGE ( 'NONE', *, *, #11204, .T. ) ;
#11734=ADVANCED_FACE ( 'NONE', ( #35663, #25639 ), #15622, .F. ) ;
#11735=EDGE_CURVE ( 'NONE', #12494, #21058, #6271, .T. ) ;
#11736=ORIENTED_EDGE ( 'NONE', *, *, #738, .F. ) ;
#11738=VERTEX_POINT ( 'NONE', #18818 ) ;
#11741=PRESENTATION_STYLE_ASSIGNMENT (( #40933 ) ) ;
#11750=ORIENTED_EDGE ( 'NONE', *, *, #10911, .F. ) ;
#11752=DIRECTION ( 'NONE',  ( -1.000000000000000000, 0.000000000000000000, 0.000000000000000000 ) ) ;
#11759=AXIS2_PLACEMENT_3D ( 'NONE', #40441, #15682, #34457 ) ;
#11767=DIRECTION ( 'NONE',  ( -1.000000000000000000, 0.000000000000000000, 0.000000000000000000 ) ) ;
#11770=CARTESIAN_POINT ( 'NONE',  ( 18.13811525448111439, 9.293884745518885993, 0.000000000000000000 ) ) ;
#11777=LINE ( 'NONE', #20727, #41689 ) ;
#11807=CONICAL_SURFACE ( 'NONE', #20647, 13.46199999999999619, 0.7853981633974497223 ) ;
#11810=DIRECTION ( 'NONE',  ( -1.000000000000000000, 0.000000000000000000, 0.000000000000000000 ) ) ;
#11811=EDGE_CURVE ( 'NONE', #15919, #11643, #35875, .T. ) ;
#11813=ORIENTED_EDGE ( 'NONE', *, *, #12782, .F. ) ;
#11825=AXIS2_PLACEMENT_3D ( 'NONE', #39426, #32606, #29409 ) ;
#11826=ORIENTED_EDGE ( 'NONE', *, *, #3029, .F. ) ;
#11832=DIRECTION ( 'NONE',  ( 9.627370216492862708E-17, 1.000000000000000000, -0.000000000000000000 ) ) ;
#11856=LINE ( 'NONE', #15251, #41751 ) ;
#11869=CARTESIAN_POINT ( 'NONE',  ( 5.223971174379742344, 56.51500000000003610, -4.542495777410184843 ) ) ;
#11876=ORIENTED_EDGE ( 'NONE', *, *, #41268, .T. ) ;
#11914=PLANE ( 'NONE',  #4858 ) ;
#11919=CARTESIAN_POINT ( 'NONE',  ( 12.21488373879589240, 17.14499999999999957, 5.016499999999999737 ) ) ;
#11957=CARTESIAN_POINT ( 'NONE',  ( 12.87096146653068196, 58.93153423982063543, -10.60403923708992835 ) ) ;
#11961=ORIENTED_EDGE ( 'NONE', *, *, #16452, .F. ) ;
#11985=EDGE_LOOP ( 'NONE', ( #20643, #32853, #16744, #747, #2754, #29009, #28759, #26268, #32504, #18155 ) ) ;
#11997=VERTEX_POINT ( 'NONE', #28988 ) ;
#12002=AXIS2_PLACEMENT_3D ( 'NONE', #4505, #10240, #20657 ) ;
#12015=CARTESIAN_POINT ( 'NONE',  ( -19.68500000000000227, 71.11999999999999034, 1.904999999999987592 ) ) ;
#12022=DIRECTION ( 'NONE',  ( -0.000000000000000000, -1.000000000000000000, -0.000000000000000000 ) ) ;
#12026=CARTESIAN_POINT ( 'NONE',  ( -5.664977208693889210, 53.58606249999999704, -5.033228321271210781 ) ) ;
#12028=EDGE_CURVE ( 'NONE', #22529, #11997, #9609, .T. ) ;
#12033=PLANE ( 'NONE',  #31227 ) ;
#12044=CARTESIAN_POINT ( 'NONE',  ( -17.14499999999999957, 71.11999999999999034, 5.016499999999999737 ) ) ;
#12048=CARTESIAN_POINT ( 'NONE',  ( -5.938381009910493447, 56.51499999999998636, -4.381499999999999950 ) ) ;
#12066=ADVANCED_FACE ( 'NONE', ( #15578 ), #38392, .T. ) ;
#12078=CARTESIAN_POINT ( 'NONE',  ( 5.224225543104745739, 57.15000000000486580, -5.327462464253549079 ) ) ;
#12080=CARTESIAN_POINT ( 'NONE',  ( 6.266702236064160658, 78.85741254032750192, 4.063604302808982105 ) ) ;
#12092=ORIENTED_EDGE ( 'NONE', *, *, #27688, .F. ) ;
#12096=CARTESIAN_POINT ( 'NONE',  ( 5.653927021192486357, 78.90752773945908416, -4.880377097574617906 ) ) ;
#12100=ADVANCED_FACE ( 'NONE', ( #29198 ), #12399, .T. ) ;
#12121=ORIENTED_EDGE ( 'NONE', *, *, #2518, .F. ) ;
#12124=CARTESIAN_POINT ( 'NONE',  ( 5.460472493305315922, 56.51499999999995794, 4.448254263655320173 ) ) ;
#12125=EDGE_CURVE ( 'NONE', #22885, #28739, #26700, .T. ) ;
#12137=AXIS2_PLACEMENT_3D ( 'NONE', #3392, #35974, #16358 ) ;
#12141=DIRECTION ( 'NONE',  ( 0.000000000000000000, 1.000000000000000000, 0.000000000000000000 ) ) ;
#12144=DIRECTION ( 'NONE',  ( -1.000000000000000000, -1.092739197465705287E-15, 0.000000000000000000 ) ) ;
#12178=VECTOR ( 'NONE', #1833, 1000.000000000000000 ) ;
#12179=AXIS2_PLACEMENT_3D ( 'NONE', #19196, #6225, #12604 ) ;
#12181=B_SPLINE_CURVE_WITH_KNOTS ( 'NONE', 3,
 ( #24971, #4981, #30941, #8366 ),
 .UNSPECIFIED., .F., .F.,
 ( 4, 4 ),
 ( 0.000000000000000000, 0.9716004430332778607 ),
 .UNSPECIFIED. ) ;
#12191=CARTESIAN_POINT ( 'NONE',  ( -5.736468567008435215, 78.90050738914777639, -5.037638016205330693 ) ) ;
#12225=ORIENTED_EDGE ( 'NONE', *, *, #6639, .T. ) ;
#12238=ORIENTED_EDGE ( 'NONE', *, *, #30280, .T. ) ;
#12263=AXIS2_PLACEMENT_3D ( 'NONE', #32826, #22361, #32192 ) ;
#12264=DIRECTION ( 'NONE',  ( -0.000000000000000000, 1.000000000000000000, -0.000000000000000000 ) ) ;
#12302=CARTESIAN_POINT ( 'NONE',  ( 10.28897677580358305, 57.14999999999999858, -5.016499999999999737 ) ) ;
#12310=CARTESIAN_POINT ( 'NONE',  ( 6.756648348127327175, 78.81597664337223819, -3.183520453979959086 ) ) ;
#12331=ADVANCED_FACE ( 'NONE', ( #20806 ), #4660, .F. ) ;
#12341=LINE ( 'NONE', #8727, #41091 ) ;
#12342=VECTOR ( 'NONE', #10600, 1000.000000000000000 ) ;
#12344=CARTESIAN_POINT ( 'NONE',  ( 5.506767014370323565, 78.91949168437542994, 5.113098386149627750 ) ) ;
#12347=CARTESIAN_POINT ( 'NONE',  ( -6.059261036834473479, 56.81853847168529370, -4.948064083792231393 ) ) ;
#12351=CYLINDRICAL_SURFACE ( 'NONE', #17975, 6.350000000000004974 ) ;
#12352=EDGE_CURVE ( 'NONE', #24559, #29906, #27426, .T. ) ;
#12360=ADVANCED_FACE ( 'NONE', ( #19601 ), #40439, .T. ) ;
#12369=EDGE_LOOP ( 'NONE', ( #37068, #4093, #15904, #5156, #29309, #26333, #22301, #2934 ) ) ;
#12373=AXIS2_PLACEMENT_3D ( 'NONE', #2776, #14893, #15732 ) ;
#12396=CARTESIAN_POINT ( 'NONE',  ( -13.85159022459153988, 16.51000000000000156, 5.016499999999999737 ) ) ;
#12399=CYLINDRICAL_SURFACE ( 'NONE', #23265, 6.350000000000004974 ) ;
#12410=LINE ( 'NONE', #2628, #26319 ) ;
#12412=ADVANCED_FACE ( 'NONE', ( #4453 ), #3445, .F. ) ;
#12419=VERTEX_POINT ( 'NONE', #21018 ) ;
#12450=DIRECTION ( 'NONE',  ( 9.627370216492862708E-17, 1.000000000000000000, -0.000000000000000000 ) ) ;
#12458=CARTESIAN_POINT ( 'NONE',  ( -5.664977208693889210, 65.30181249999998272, -5.033228321271210781 ) ) ;
#12470=CARTESIAN_POINT ( 'NONE',  ( 5.749535644242491195, 78.89971493812817016, -5.036102041843245836 ) ) ;
#12471=CIRCLE ( 'NONE', #41053, 0.6350000000000001199 ) ;
#12478=CARTESIAN_POINT ( 'NONE',  ( -5.266289895157169814E-14, 83.56599999999998829, 1.904999999999999805 ) ) ;
#12491=AXIS2_PLACEMENT_3D ( 'NONE', #17584, #33592, #4425 ) ;
#12493=AXIS2_PLACEMENT_3D ( 'NONE', #15038, #24625, #37839 ) ;
#12494=VERTEX_POINT ( 'NONE', #34041 ) ;
#12519=CARTESIAN_POINT ( 'NONE',  ( -14.39766717389552575, 60.87500489999897013, 1.905000000000008464 ) ) ;
#12539=ORIENTED_EDGE ( 'NONE', *, *, #18005, .T. ) ;
#12542=CARTESIAN_POINT ( 'NONE',  ( 20.83467972660109169, 65.95194780259438971, 5.016499999999999737 ) ) ;
#12554=ORIENTED_EDGE ( 'NONE', *, *, #15522, .T. ) ;
#12567=ADVANCED_FACE ( 'NONE', ( #26802 ), #14006, .F. ) ;
#12570=CARTESIAN_POINT ( 'NONE',  ( 5.938360781727902271, 56.51500000000000057, -4.381499999999999062 ) ) ;
#12593=ORIENTED_EDGE ( 'NONE', *, *, #12597, .T. ) ;
#12594=DIRECTION ( 'NONE',  ( 6.353134868986659519E-16, -1.000000000000000000, 0.000000000000000000 ) ) ;
#12595=ADVANCED_FACE ( 'NONE', ( #14211 ), #34222, .F. ) ;
#12596=CYLINDRICAL_SURFACE ( 'NONE', #11639, 6.350000000000004974 ) ;
#12597=EDGE_CURVE ( 'NONE', #7919, #20294, #37029, .T. ) ;
#12604=DIRECTION ( 'NONE',  ( -1.000000000000000000, 1.288607544181256449E-16, 0.000000000000000000 ) ) ;
#12611=CARTESIAN_POINT ( 'NONE',  ( 19.68500000000000227, 71.11999999999999034, 5.016499999999999737 ) ) ;
#12621=CARTESIAN_POINT ( 'NONE',  ( 5.965356522962838248, 77.01756249999996840, 5.016499999999999737 ) ) ;
#12661=DIRECTION ( 'NONE',  ( 9.627370216492862708E-17, 1.000000000000000000, -0.000000000000000000 ) ) ;
#12675=CARTESIAN_POINT ( 'NONE',  ( 5.787341484272322312, 78.89667267365581438, -5.030122981225435552 ) ) ;
#12682=DIRECTION ( 'NONE',  ( -0.000000000000000000, -1.000000000000000000, -0.000000000000000000 ) ) ;
#12695=ADVANCED_FACE ( 'NONE', ( #25063 ), #8675, .T. ) ;
#12698=EDGE_CURVE ( 'NONE', #4024, #35923, #37428, .T. ) ;
#12708=B_SPLINE_CURVE_WITH_KNOTS ( 'NONE', 3,
 ( #41243, #12048, #2057, #8649, #21610, #40823 ),
 .UNSPECIFIED., .F., .F.,
 ( 4, 2, 4 ),
 ( 0.000000000000000000, 0.0003611586812565052425, 0.0007223173625130104849 ),
 .UNSPECIFIED. ) ;
#12713=ORIENTED_EDGE ( 'NONE', *, *, #7093, .T. ) ;
#12719=ORIENTED_EDGE ( 'NONE', *, *, #8174, .T. ) ;
#12723=CARTESIAN_POINT ( 'NONE',  ( -6.057513928997640740, 57.78499999999998948, 1.905000000000003579 ) ) ;
#12730=CARTESIAN_POINT ( 'NONE',  ( -9.925711944554160837, 78.55658865046541450, 5.016499999999999737 ) ) ;
#12739=AXIS2_PLACEMENT_3D ( 'NONE', #41882, #19058, #22448 ) ;
#12746=DIRECTION ( 'NONE',  ( 0.000000000000000000, -1.000000000000000000, 0.000000000000000000 ) ) ;
#12751=FACE_OUTER_BOUND ( 'NONE', #4755, .T. ) ;
#12758=ORIENTED_EDGE ( 'NONE', *, *, #27726, .T. ) ;
#12759=CARTESIAN_POINT ( 'NONE',  ( -5.177913976931290740, 64.41499993257282597, 5.372100000000001430 ) ) ;
#12772=CARTESIAN_POINT ( 'NONE',  ( 12.21488373879589240, 55.24500000000000455, -5.016499999999999737 ) ) ;
#12775=ORIENTED_EDGE ( 'NONE', *, *, #25053, .F. ) ;
#12781=ORIENTED_EDGE ( 'NONE', *, *, #2707, .F. ) ;
#12782=EDGE_CURVE ( 'NONE', #35912, #19939, #18764, .T. ) ;
#12783=ORIENTED_EDGE ( 'NONE', *, *, #8517, .F. ) ;
#12805=LINE ( 'NONE', #6428, #37325 ) ;
#12814=VECTOR ( 'NONE', #7908, 1000.000000000000000 ) ;
#12819=CARTESIAN_POINT ( 'NONE',  ( -14.80692295515835255, 78.04183178746349370, -5.016499999999999737 ) ) ;
#12825=CARTESIAN_POINT ( 'NONE',  ( 5.871452009091292723, 77.01756249999996840, 5.016499999999999737 ) ) ;
#12845=ORIENTED_EDGE ( 'NONE', *, *, #7939, .F. ) ;
#12855=CARTESIAN_POINT ( 'NONE',  ( -14.39766717389551687, 57.78499999999998948, -1.905000000000000027 ) ) ;
#12874=EDGE_CURVE ( 'NONE', #12419, #41231, #16192, .T. ) ;
#12888=PLANE ( 'NONE',  #18647 ) ;
#12899=AXIS2_PLACEMENT_3D ( 'NONE', #32295, #16085, #29937 ) ;
#12902=AXIS2_PLACEMENT_3D ( 'NONE', #19730, #25922, #38719 ) ;
#12904=LINE ( 'NONE', #13118, #16557 ) ;
#12908=CARTESIAN_POINT ( 'NONE',  ( -4.897655256226316034, 56.53910281269282478, 5.081330806033710346 ) ) ;
#12914=LINE ( 'NONE', #13131, #41023 ) ;
#12920=VERTEX_POINT ( 'NONE', #19430 ) ;
#12925=CARTESIAN_POINT ( 'NONE',  ( 13.17422243436029916, 17.14500000000093394, 5.016499999999999737 ) ) ;
#12927=EDGE_CURVE ( 'NONE', #11069, #11444, #25206, .T. ) ;
#12931=LINE ( 'NONE', #32113, #39157 ) ;
#12945=CARTESIAN_POINT ( 'NONE',  ( -23.49500000000000455, 71.11999999999999034, 5.016499999999999737 ) ) ;
#12964=DIRECTION ( 'NONE',  ( -1.000000000000000000, 0.000000000000000000, 0.000000000000000000 ) ) ;
#12969=DIRECTION ( 'NONE',  ( -5.463695987328526437E-16, -1.000000000000000000, -1.672774450599033775E-31 ) ) ;
#12973=CARTESIAN_POINT ( 'NONE',  ( 14.39766717389552042, 60.02151067229126369, -1.904999999999999583 ) ) ;
#12976=SURFACE_STYLE_FILL_AREA ( #19158 ) ;
#12998=CIRCLE ( 'NONE', #19131, 16.60960244842765832 ) ;
#13002=ORIENTED_EDGE ( 'NONE', *, *, #27922, .T. ) ;
#13033=CARTESIAN_POINT ( 'NONE',  ( 5.241362157049057835, 65.30181249999998272, 5.310945289804168468 ) ) ;
#13067=CIRCLE ( 'NONE', #11703, 0.6350000000000001199 ) ;
#13074=CARTESIAN_POINT ( 'NONE',  ( -5.241362157049148429, 88.73331249999998249, 5.310945289804168468 ) ) ;
#13085=DIRECTION ( 'NONE',  ( 1.000000000000000000, -9.627370216492862708E-17, 0.000000000000000000 ) ) ;
#13101=ORIENTED_EDGE ( 'NONE', *, *, #7093, .F. ) ;
#13102=DIRECTION ( 'NONE',  ( 1.000000000000000000, 0.000000000000000000, 0.000000000000000000 ) ) ;
#13118=CARTESIAN_POINT ( 'NONE',  ( -11.58677707360137532, 12.96416000000000146, -4.474811398758259173 ) ) ;
#13131=CARTESIAN_POINT ( 'NONE',  ( -13.85159022459153988, 71.11999999999999034, -5.016499999999999737 ) ) ;
#13136=VERTEX_POINT ( 'NONE', #22672 ) ;
#13147=CARTESIAN_POINT ( 'NONE',  ( 10.92199999999999704, 16.51000000000000156, 0.000000000000000000 ) ) ;
#13152=CARTESIAN_POINT ( 'NONE',  ( 4.737240446979624764, 56.51500000000001478, 4.914899999999992275 ) ) ;
#13154=AXIS2_PLACEMENT_3D ( 'NONE', #21441, #21238, #2098 ) ;
#13157=EDGE_LOOP ( 'NONE', ( #35853, #40144 ) ) ;
#13164=AXIS2_PLACEMENT_3D ( 'NONE', #32664, #35660, #38436 ) ;
#13168=CARTESIAN_POINT ( 'NONE',  ( 9.094996104468812348, 78.64197151092923832, 1.904999999999988258 ) ) ;
#13178=PLANE ( 'NONE',  #12137 ) ;
#13180=CARTESIAN_POINT ( 'NONE',  ( 14.39766717389552220, 57.78500000000000369, 1.904999999999991367 ) ) ;
#13194=CARTESIAN_POINT ( 'NONE',  ( 14.79536922792820697, 61.64024183321802042, -1.904999999999999583 ) ) ;
#13203=EDGE_LOOP ( 'NONE', ( #27815, #18339, #10998, #3684, #7731 ) ) ;
#13205=AXIS2_PLACEMENT_3D ( 'NONE', #33252, #14056, #27061 ) ;
#13222=LINE ( 'NONE', #35381, #18813 ) ;
#13227=CARTESIAN_POINT ( 'NONE',  ( -6.059261036834476144, 57.14999999999999858, -5.016499999999999737 ) ) ;
#13228=DIRECTION ( 'NONE',  ( 1.000000000000000000, 0.000000000000000000, 0.000000000000000000 ) ) ;
#13229=CARTESIAN_POINT ( 'NONE',  ( 14.60500000000000043, 71.11999999999999034, 5.016499999999999737 ) ) ;
#13262=DIRECTION ( 'NONE',  ( 9.627370216492862708E-17, 1.000000000000000000, -0.000000000000000000 ) ) ;
#13274=CARTESIAN_POINT ( 'NONE',  ( 11.58677707360137532, 17.14499999999999957, -4.474811398758258285 ) ) ;
#13275=DIRECTION ( 'NONE',  ( 0.000000000000000000, 1.000000000000000000, 0.000000000000000000 ) ) ;
#13289=CARTESIAN_POINT ( 'NONE',  ( -5.965356522962950159, 77.01756250000002524, 5.016499999999999737 ) ) ;
#13298=ORIENTED_EDGE ( 'NONE', *, *, #38651, .F. ) ;
#13310=DIRECTION ( 'NONE',  ( 0.000000000000000000, 0.000000000000000000, 1.000000000000000000 ) ) ;
#13314=ORIENTED_EDGE ( 'NONE', *, *, #19110, .F. ) ;
#13334=DIRECTION ( 'NONE',  ( 1.000000000000000000, 6.353134868986659519E-16, -0.000000000000000000 ) ) ;
#13352=ORIENTED_EDGE ( 'NONE', *, *, #23772, .F. ) ;
#13356=CARTESIAN_POINT ( 'NONE',  ( 13.17422243436029916, 17.14500000000093394, 5.016499999999999737 ) ) ;
#13384=CARTESIAN_POINT ( 'NONE',  ( -5.322370863981875644, 57.14999999999976410, -5.239063870260801004 ) ) ;
#13417=CIRCLE ( 'NONE', #12739, 0.6350000000000001199 ) ;
#13421=EDGE_LOOP ( 'NONE', ( #1052, #39524, #39947, #15065 ) ) ;
#13430=EDGE_CURVE ( 'NONE', #1544, #32690, #28153, .T. ) ;
#13438=FACE_OUTER_BOUND ( 'NONE', #11280, .T. ) ;
#13444=CARTESIAN_POINT ( 'NONE',  ( 8.515285667870289099E-16, 8.844871939465425825, 0.000000000000000000 ) ) ;
#13453=CARTESIAN_POINT ( 'NONE',  ( -17.14499999999999957, 71.11999999999999034, -5.016499999999999737 ) ) ;
#13458=CARTESIAN_POINT ( 'NONE',  ( 1.650612623617701257E-15, 17.14499999999999957, 0.000000000000000000 ) ) ;
#13473=ORIENTED_EDGE ( 'NONE', *, *, #24839, .T. ) ;
#13478=LINE ( 'NONE', #30496, #4186 ) ;
#13484=ORIENTED_EDGE ( 'NONE', *, *, #15651, .T. ) ;
#13487=EDGE_LOOP ( 'NONE', ( #19062, #24410, #18836, #16862 ) ) ;
#13505=CARTESIAN_POINT ( 'NONE',  ( -5.241362157049148429, 77.01756250000002524, 5.310945289804168468 ) ) ;
#13506=CARTESIAN_POINT ( 'NONE',  ( -6.059261036834477032, 57.14999999999997726, 5.016499999999999737 ) ) ;
#13547=CARTESIAN_POINT ( 'NONE',  ( -17.14499999999999957, 71.11999999999999034, 5.016499999999999737 ) ) ;
#13555=EDGE_CURVE ( 'NONE', #32240, #33599, #19741, .T. ) ;
#13560=VERTEX_POINT ( 'NONE', #4924 ) ;
#13566=CARTESIAN_POINT ( 'NONE',  ( 7.213960532363566713, 83.56599999999998829, -1.904999999999999805 ) ) ;
#13579=CARTESIAN_POINT ( 'NONE',  ( 5.813542725970706648, 56.51499999999999346, 4.384680539058527948 ) ) ;
#13590=CARTESIAN_POINT ( 'NONE',  ( -9.094996104468895837, 78.64197151092922411, 1.904999999999988258 ) ) ;
#13600=LINE ( 'NONE', #24805, #23000 ) ;
#13606=ORIENTED_EDGE ( 'NONE', *, *, #36604, .F. ) ;
#13608=( BOUNDED_SURFACE ( )  B_SPLINE_SURFACE ( 3, 2, ( 
 ( #21639, #1876, #41273 ),
 ( #34664, #38284, #28050 ),
 ( #37430, #2302, #25279 ),
 ( #41059, #28685, #34253 ),
 ( #5917, #31241, #41485 ),
 ( #11869, #11652, #31036 ),
 ( #2085, #24859, #31675 ),
 ( #37855, #5492, #2724 ),
 ( #18453, #31458, #15262 ),
 ( #9103, #28266, #8886 ),
 ( #22068, #35095, #12078 ),
 ( #34879, #18879, #35723 ) ),
 .UNSPECIFIED., .F., .F., .T. ) 
 B_SPLINE_SURFACE_WITH_KNOTS ( ( 4, 2, 2, 2, 2, 4 ),
 ( 3, 3 ),
 ( 0.000000000000000000, 0.0003677900075225773967, 0.0007355800150451547934, 0.001103370022567732190, 0.001287265026329020888, 0.001471160030090309587 ),
 ( 0.000000000000000000, 1.000000000000000000 ),
 .UNSPECIFIED. ) 
 GEOMETRIC_REPRESENTATION_ITEM ( )  RATIONAL_B_SPLINE_SURFACE ( (
 ( 1.000000000000000000, 0.7071067811865475727, 1.000000000000000000),
 ( 1.000000000000000000, 0.7071067811865475727, 1.000000000000000000),
 ( 1.000000000000000000, 0.7071067811865552333, 1.000000000000000000),
 ( 1.000000000000000000, 0.7071067811865552333, 1.000000000000000000),
 ( 1.000000000000000000, 0.7071067811865553443, 1.000000000000000000),
 ( 1.000000000000000000, 0.7071067811865553443, 1.000000000000000000),
 ( 1.000000000000000000, 0.7071067811865398012, 1.000000000000000000),
 ( 1.000000000000000000, 0.7071067811865398012, 1.000000000000000000),
 ( 1.000000000000000000, 0.7071067811865514585, 1.000000000000000000),
 ( 1.000000000000000000, 0.7071067811865514585, 1.000000000000000000),
 ( 1.000000000000000000, 0.7071067811865514585, 1.000000000000000000),
 ( 1.000000000000000000, 0.7071067811865514585, 1.000000000000000000) ) ) 
 REPRESENTATION_ITEM ( '' )  SURFACE ( )  );
#13640=ORIENTED_EDGE ( 'NONE', *, *, #30481, .T. ) ;
#13648=ADVANCED_FACE ( 'NONE', ( #30462 ), #1307, .T. ) ;
#13650=AXIS2_PLACEMENT_3D ( 'NONE', #33043, #16837, #29837 ) ;
#13653=CARTESIAN_POINT ( 'NONE',  ( 11.82906070755491434, 56.41571150956137615, 5.016499999999999737 ) ) ;
#13661=PLANE ( 'NONE',  #5936 ) ;
#13672=CARTESIAN_POINT ( 'NONE',  ( -6.059261036834476144, 56.51499999999998636, 4.381499999999999950 ) ) ;
#13688=CIRCLE ( 'NONE', #16368, 6.350000000000004974 ) ;
#13713=CARTESIAN_POINT ( 'NONE',  ( -5.475330206976889436, 88.73331249999998249, 5.107412922131463695 ) ) ;
#13726=AXIS2_PLACEMENT_3D ( 'NONE', #14955, #21757, #8582 ) ;
#13734=CARTESIAN_POINT ( 'NONE',  ( 6.059261036834400649, 64.39150124418098642, 5.016499999999999737 ) ) ;
#13735=LINE ( 'NONE', #33552, #5755 ) ;
#13757=CARTESIAN_POINT ( 'NONE',  ( 14.73199999999999932, 57.78500000000000369, 0.000000000000000000 ) ) ;
#13799=LINE ( 'NONE', #40017, #12342 ) ;
#13821=AXIS2_PLACEMENT_3D ( 'NONE', #16598, #33020, #3003 ) ;
#13832=CARTESIAN_POINT ( 'NONE',  ( 5.664977208693799504, 88.73331249999999670, -5.033228321271210781 ) ) ;
#13856=CARTESIAN_POINT ( 'NONE',  ( -12.21488373879589240, 55.24499999999999034, 5.016499999999999737 ) ) ;
#13858=( BOUNDED_SURFACE ( )  B_SPLINE_SURFACE ( 3, 2, ( 
 ( #23064, #6911, #13506 ),
 ( #15684, #25285, #26066 ),
 ( #10305, #7129, #20085 ),
 ( #9107, #3939, #739 ),
 ( #38076, #34883, #5715 ),
 ( #38288, #22071, #35098 ),
 ( #4362, #20289, #7958 ),
 ( #950, #23485, #36933 ),
 ( #14122, #4781, #39714 ),
 ( #17730, #7541, #13919 ),
 ( #27335, #27121, #40554 ),
 ( #10928, #7753, #33949 ) ),
 .UNSPECIFIED., .F., .F., .F. ) 
 B_SPLINE_SURFACE_WITH_KNOTS ( ( 4, 2, 2, 2, 2, 4 ),
 ( 3, 3 ),
 ( -1.734723475976807094E-18, 0.0003677900075225834682, 0.0007355800150451686711, 0.001103370022567753874, 0.001287265026329046476, 0.001471160030090339077 ),
 ( 0.000000000000000000, 1.000000000000000000 ),
 .UNSPECIFIED. ) 
 GEOMETRIC_REPRESENTATION_ITEM ( )  RATIONAL_B_SPLINE_SURFACE ( (
 ( 1.000000000000000000, 0.7071067811865475727, 1.000000000000000000),
 ( 1.000000000000000000, 0.7071067811865475727, 1.000000000000000000),
 ( 1.000000000000000000, 0.7071067811865514585, 1.000000000000000000),
 ( 1.000000000000000000, 0.7071067811865514585, 1.000000000000000000),
 ( 1.000000000000000000, 0.7071067811865436870, 1.000000000000000000),
 ( 1.000000000000000000, 0.7071067811865436870, 1.000000000000000000),
 ( 1.000000000000000000, 0.7071067811865514585, 1.000000000000000000),
 ( 1.000000000000000000, 0.7071067811865514585, 1.000000000000000000),
 ( 1.000000000000000000, 0.7071067811865514585, 1.000000000000000000),
 ( 1.000000000000000000, 0.7071067811865514585, 1.000000000000000000),
 ( 1.000000000000000000, 0.7071067811865475727, 1.000000000000000000),
 ( 1.000000000000000000, 0.7071067811865475727, 1.000000000000000000) ) ) 
 REPRESENTATION_ITEM ( '' )  SURFACE ( )  );
#13862=CARTESIAN_POINT ( 'NONE',  ( 11.62920297224753874, 55.59919541885984273, 5.016499999999892268 ) ) ;
#13871=CARTESIAN_POINT ( 'NONE',  ( -5.525651935317164920, 78.91763798174274314, 5.107334513333068315 ) ) ;
#13894=EDGE_CURVE ( 'NONE', #4862, #9633, #12341, .T. ) ;
#13904=CARTESIAN_POINT ( 'NONE',  ( 10.28897677580358128, 56.51500000000000057, -5.016500000000001513 ) ) ;
#13919=CARTESIAN_POINT ( 'NONE',  ( -5.256643466843552659, 57.14999999999978542, 5.296410794270378197 ) ) ;
#13924=EDGE_LOOP ( 'NONE', ( #8972, #26092, #37012, #34223, #21179, #3763, #17601, #9359, #23549 ) ) ;
#13947=EDGE_CURVE ( 'NONE', #4862, #5073, #17956, .T. ) ;
#13959=CARTESIAN_POINT ( 'NONE',  ( -14.60500000000000043, 71.11999999999999034, 5.016499999999999737 ) ) ;
#13964=DIRECTION ( 'NONE',  ( -1.000000000000000000, -6.353134868986659519E-16, 0.000000000000000000 ) ) ;
#13967=ORIENTED_EDGE ( 'NONE', *, *, #18043, .F. ) ;
#13999=ORIENTED_EDGE ( 'NONE', *, *, #5023, .T. ) ;
#14006=CYLINDRICAL_SURFACE ( 'NONE', #26741, 13.46199999999999442 ) ;
#14008=CARTESIAN_POINT ( 'NONE',  ( -14.79536922792820697, 61.64024183321802042, -1.904999999999999583 ) ) ;
#14016=VERTEX_POINT ( 'NONE', #15311 ) ;
#14024=AXIS2_PLACEMENT_3D ( 'NONE', #10889, #23876, #7714 ) ;
#14032=VECTOR ( 'NONE', #21279, 1000.000000000000000 ) ;
#14035=CARTESIAN_POINT ( 'NONE',  ( 5.871452009091292723, 88.73331249999999670, -5.016499999999999737 ) ) ;
#14042=EDGE_CURVE ( 'NONE', #25936, #33599, #17189, .T. ) ;
#14056=DIRECTION ( 'NONE',  ( -9.627370216492862708E-17, -1.000000000000000000, 0.000000000000000000 ) ) ;
#14072=DIRECTION ( 'NONE',  ( 1.000000000000000000, 0.000000000000000000, -0.000000000000000000 ) ) ;
#14076=DIRECTION ( 'NONE',  ( 9.627370216492862708E-17, 1.000000000000000000, -0.000000000000000000 ) ) ;
#14077=CARTESIAN_POINT ( 'NONE',  ( -4.968812502058939984, 56.51947257897013088, -4.801689445541318157 ) ) ;
#14085=ORIENTED_EDGE ( 'NONE', *, *, #23404, .T. ) ;
#14090=ADVANCED_FACE ( 'NONE', ( #11704 ), #41374, .T. ) ;
#14101=EDGE_CURVE ( 'NONE', #17420, #18200, #26677, .T. ) ;
#14115=EDGE_CURVE ( 'NONE', #6407, #24827, #16582, .T. ) ;
#14122=CARTESIAN_POINT ( 'NONE',  ( -4.918180946948480070, 56.51500000000000767, 4.748993904427170065 ) ) ;
#14126=ORIENTED_EDGE ( 'NONE', *, *, #32350, .F. ) ;
#14159=CARTESIAN_POINT ( 'NONE',  ( -4.897655256226337350, 56.53910281269283900, -5.081330806033717451 ) ) ;
#14166=ADVANCED_FACE ( 'NONE', ( #12751 ), #22943, .F. ) ;
#14182=CARTESIAN_POINT ( 'NONE',  ( -5.652760403059880367, 78.90762248850967353, -4.881857480398479332 ) ) ;
#14187=CARTESIAN_POINT ( 'NONE',  ( -13.85159022459153988, 60.48513866567135722, -5.016500000000000625 ) ) ;
#14188=DIRECTION ( 'NONE',  ( 0.1728608224830406603, -0.000000000000000000, -0.9849462604886047856 ) ) ;
#14204=ORIENTED_EDGE ( 'NONE', *, *, #29434, .F. ) ;
#14211=FACE_OUTER_BOUND ( 'NONE', #39905, .T. ) ;
#14215=ADVANCED_FACE ( 'NONE', ( #25945 ), #9553, .T. ) ;
#14229=CARTESIAN_POINT ( 'NONE',  ( 6.349999999999948130, 83.56599999999998829, 5.803602218936700314E-46 ) ) ;
#14239=CARTESIAN_POINT ( 'NONE',  ( 5.241362157049057835, 65.30181249999998272, -5.310945289804168468 ) ) ;
#14261=DIRECTION ( 'NONE',  ( 9.627370216492862708E-17, 1.000000000000000000, -0.000000000000000000 ) ) ;
#14262=FACE_OUTER_BOUND ( 'NONE', #9377, .T. ) ;
#14266=DIRECTION ( 'NONE',  ( 0.7071067811865465735, -0.7071067811865484609, 0.000000000000000000 ) ) ;
#14274=CARTESIAN_POINT ( 'NONE',  ( -5.632494751984450154, 78.90911215162431347, 5.063853515468840882 ) ) ;
#14275=DIRECTION ( 'NONE',  ( -1.000000000000000000, 0.000000000000000000, 0.000000000000000000 ) ) ;
#14282=CIRCLE ( 'NONE', #20385, 12.69999999999999751 ) ;
#14301=ORIENTED_EDGE ( 'NONE', *, *, #4113, .T. ) ;
#14304=FACE_OUTER_BOUND ( 'NONE', #6560, .T. ) ;
#14311=ADVANCED_FACE ( 'NONE', ( #17206 ), #20808, .T. ) ;
#14314=CARTESIAN_POINT ( 'NONE',  ( -10.28897677580358305, 56.51499999999998636, 4.381499999999999950 ) ) ;
#14330=CYLINDRICAL_SURFACE ( 'NONE', #39847, 2.540000000000000480 ) ;
#14342=ORIENTED_EDGE ( 'NONE', *, *, #19024, .F. ) ;
#14358=AXIS2_PLACEMENT_3D ( 'NONE', #19177, #5795, #32183 ) ;
#14363=VECTOR ( 'NONE', #36143, 1000.000000000000000 ) ;
#14369=CARTESIAN_POINT ( 'NONE',  ( 5.475330206976797953, 57.14999999999998437, 5.107412922131463695 ) ) ;
#14370=VECTOR ( 'NONE', #18671, 999.9999999999998863 ) ;
#14394=CARTESIAN_POINT ( 'NONE',  ( 16.60960244842765832, 17.14499999999999957, 2.034089647357696937E-15 ) ) ;
#14404=ORIENTED_EDGE ( 'NONE', *, *, #15368, .F. ) ;
#14411=ORIENTED_EDGE ( 'NONE', *, *, #37367, .F. ) ;
#14415=AXIS2_PLACEMENT_3D ( 'NONE', #26913, #35207, #5618 ) ;
#14441=ADVANCED_FACE ( 'NONE', ( #7221 ), #29992, .T. ) ;
#14442=LINE ( 'NONE', #27451, #41258 ) ;
#14446=CARTESIAN_POINT ( 'NONE',  ( 14.39766717389551864, 57.78500000000000369, -1.904999999999999583 ) ) ;
#14466=EDGE_CURVE ( 'NONE', #15919, #14963, #29665, .T. ) ;
#14470=( BOUNDED_CURVE ( )  B_SPLINE_CURVE ( 3, ( #16540, #6756, #25503, #6135 ),
 .UNSPECIFIED., .F., .F. ) 
 B_SPLINE_CURVE_WITH_KNOTS ( ( 4, 4 ),
 ( 1.570796326794894782, 2.532278806861536946 ),
 .UNSPECIFIED. ) 
 CURVE ( )  GEOMETRIC_REPRESENTATION_ITEM ( )  RATIONAL_B_SPLINE_CURVE ( ( 1.000000000000000000, 0.9244349266169026302, 0.9244349266169026302, 1.000000000000000000 ) ) 
 REPRESENTATION_ITEM ( '' )  );
#14471=DIRECTION ( 'NONE',  ( -9.627370216492862708E-17, -1.000000000000000000, 0.000000000000000000 ) ) ;
#14477=CARTESIAN_POINT ( 'NONE',  ( 11.11710224466980712, 56.30409367656758235, 5.016500000000000625 ) ) ;
#14485=CARTESIAN_POINT ( 'NONE',  ( -11.08653569745421308, 56.26057688450604388, -4.438844214435591518 ) ) ;
#14512=ADVANCED_FACE ( 'NONE', ( #7847 ), #7040, .T. ) ;
#14513=ORIENTED_EDGE ( 'NONE', *, *, #12874, .T. ) ;
#14526=B_SPLINE_CURVE_WITH_KNOTS ( 'NONE', 3,
 ( #13356, #7396, #11003, #36792, #20358, #17388 ),
 .UNSPECIFIED., .F., .F.,
 ( 4, 2, 4 ),
 ( 0.0008205648557148674267, 0.001333860798246176271, 0.001847156740777485115 ),
 .UNSPECIFIED. ) ;
#14529=CARTESIAN_POINT ( 'NONE',  ( -10.63219908769220901, 56.50600268266015291, 5.016499999998452530 ) ) ;
#14538=FACE_OUTER_BOUND ( 'NONE', #30739, .T. ) ;
#14545=EDGE_LOOP ( 'NONE', ( #29352, #24019, #1029, #23087 ) ) ;
#14546=DIRECTION ( 'NONE',  ( -9.627370216492862708E-17, -1.000000000000000000, 0.000000000000000000 ) ) ;
#14556=CARTESIAN_POINT ( 'NONE',  ( 6.059261036834407754, 56.58343591620776891, 4.712961528314683513 ) ) ;
#14562=B_SPLINE_CURVE_WITH_KNOTS ( 'NONE', 5,
 ( #17481, #30478, #14905, #28334, #35155, #18729, #28751, #31739 ),
 .UNSPECIFIED., .F., .F.,
 ( 6, 2, 6 ),
 ( -5.999999999880332237E-08, 0.0004919218780628848613, 0.0009839037561257684989 ),
 .UNSPECIFIED. ) ;
#14568=AXIS2_PLACEMENT_3D ( 'NONE', #32918, #12682, #13310 ) ;
#14571=LINE ( 'NONE', #25008, #40201 ) ;
#14583=ORIENTED_EDGE ( 'NONE', *, *, #33678, .F. ) ;
#14592=CARTESIAN_POINT ( 'NONE',  ( 5.600204413206903986, 78.91171765783749947, -5.075433163388857416 ) ) ;
#14600=ORIENTED_EDGE ( 'NONE', *, *, #41193, .F. ) ;
#14645=ORIENTED_EDGE ( 'NONE', *, *, #8517, .T. ) ;
#14650=DIRECTION ( 'NONE',  ( 5.463695987328526437E-16, -1.000000000000000000, -1.672774450599033775E-31 ) ) ;
#14654=LINE ( 'NONE', #17438, #17797 ) ;
#14661=ORIENTED_EDGE ( 'NONE', *, *, #22509, .T. ) ;
#14663=CIRCLE ( 'NONE', #26936, 6.349999999999999645 ) ;
#14669=ORIENTED_EDGE ( 'NONE', *, *, #20953, .F. ) ;
#14675=CARTESIAN_POINT ( 'NONE',  ( 13.85159022459153988, 59.63164443796365077, -5.016499999999999737 ) ) ;
#14678=ADVANCED_FACE ( 'NONE', ( #37648 ), #18668, .F. ) ;
#14680=ADVANCED_FACE ( 'NONE', ( #38070 ), #13608, .T. ) ;
#14687=VERTEX_POINT ( 'NONE', #39335 ) ;
#14693=CARTESIAN_POINT ( 'NONE',  ( -12.21488373879589062, 55.24499999999998323, -5.016499999999999737 ) ) ;
#14711=ORIENTED_EDGE ( 'NONE', *, *, #14926, .F. ) ;
#14714=FILL_AREA_STYLE ('',( #1755 ) ) ;
#14716=DIRECTION ( 'NONE',  ( 0.7071067811865483499, -0.7071067811865465735, 0.000000000000000000 ) ) ;
#14717=( BOUNDED_CURVE ( )  B_SPLINE_CURVE ( 3, ( #16545, #23126, #14187, #7197 ),
 .UNSPECIFIED., .F., .T. ) 
 B_SPLINE_CURVE_WITH_KNOTS ( ( 4, 4 ),
 ( 1.570796326794895670, 2.532278806861539611 ),
 .UNSPECIFIED. ) 
 CURVE ( )  GEOMETRIC_REPRESENTATION_ITEM ( )  RATIONAL_B_SPLINE_CURVE ( ( 1.000000000000000000, 0.9244349266169025192, 0.9244349266169025192, 1.000000000000000000 ) ) 
 REPRESENTATION_ITEM ( '' )  );
#14721=CARTESIAN_POINT ( 'NONE',  ( -18.32410244842765934, 17.14500000000000313, 0.000000000000000000 ) ) ;
#14726=ORIENTED_EDGE ( 'NONE', *, *, #12028, .T. ) ;
#14741=CARTESIAN_POINT ( 'NONE',  ( 17.14499999999999957, 71.11999999999999034, -5.016499999999999737 ) ) ;
#14772=B_SPLINE_CURVE_WITH_KNOTS ( 'NONE', 5,
 ( #36448, #40285, #11077, #5332, #41106, #27679, #5538, #24686 ),
 .UNSPECIFIED., .F., .F.,
 ( 6, 2, 6 ),
 ( 0.000000000000000000, 0.0004921095964230306607, 0.0009842191928460613214 ),
 .UNSPECIFIED. ) ;
#14798=ORIENTED_EDGE ( 'NONE', *, *, #14466, .F. ) ;
#14803=ADVANCED_FACE ( 'NONE', ( #373 ), #38912, .T. ) ;
#14811=ORIENTED_EDGE ( 'NONE', *, *, #2912, .F. ) ;
#14812=CARTESIAN_POINT ( 'NONE',  ( 1.248107678658480997E-15, 12.96416000000000146, 0.000000000000000000 ) ) ;
#14826=CARTESIAN_POINT ( 'NONE',  ( 20.83467972660109524, 65.95194780259438971, -1.904999999999999583 ) ) ;
#14841=EDGE_CURVE ( 'NONE', #21058, #42038, #12914, .T. ) ;
#14853=FACE_OUTER_BOUND ( 'NONE', #16533, .T. ) ;
#14868=AXIS2_PLACEMENT_3D ( 'NONE', #12044, #25033, #38036 ) ;
#14893=DIRECTION ( 'NONE',  ( -0.1715592850456333085, -0.1224830539174543292, -0.9775302108976914317 ) ) ;
#14905=CARTESIAN_POINT ( 'NONE',  ( -5.305748947172282293, 57.14999999999997016, -5.247078976224250013 ) ) ;
#14926=EDGE_CURVE ( 'NONE', #8022, #33026, #17868, .T. ) ;
#14932=DIRECTION ( 'NONE',  ( -1.000000000000000000, -0.000000000000000000, -0.000000000000000000 ) ) ;
#14952=LINE ( 'NONE', #5399, #8758 ) ;
#14955=CARTESIAN_POINT ( 'NONE',  ( 17.14499999999999957, 71.11999999999999034, -5.016499999999999737 ) ) ;
#14963=VERTEX_POINT ( 'NONE', #6963 ) ;
#15000=TOROIDAL_SURFACE ( 'NONE', #17740, 17.68910244842765778, 0.6350000000000000089 ) ;
#15005=ORIENTED_EDGE ( 'NONE', *, *, #6873, .F. ) ;
#15038=CARTESIAN_POINT ( 'NONE',  ( 1.247998466936323035E-15, 12.96302561210691806, 0.000000000000000000 ) ) ;
#15040=ORIENTED_EDGE ( 'NONE', *, *, #31380, .F. ) ;
#15046=DIRECTION ( 'NONE',  ( -0.1469470846586743706, 0.000000000000000000, 0.9891443546370348727 ) ) ;
#15051=AXIS2_PLACEMENT_3D ( 'NONE', #27749, #17526, #40759 ) ;
#15056=ORIENTED_EDGE ( 'NONE', *, *, #34053, .F. ) ;
#15064=DIRECTION ( 'NONE',  ( -1.000000000000000000, 0.000000000000000000, 0.000000000000000000 ) ) ;
#15065=ORIENTED_EDGE ( 'NONE', *, *, #26982, .F. ) ;
#15086=ORIENTED_EDGE ( 'NONE', *, *, #4976, .T. ) ;
#15089=ORIENTED_EDGE ( 'NONE', *, *, #30807, .T. ) ;
#15092=ORIENTED_EDGE ( 'NONE', *, *, #5930, .F. ) ;
#15102=CARTESIAN_POINT ( 'NONE',  ( -17.14499999999999957, 71.11999999999999034, -5.016499999999999737 ) ) ;
#15113=CARTESIAN_POINT ( 'NONE',  ( 11.66725022231030984, 17.14499999999999957, -5.016499999999999737 ) ) ;
#15114=DIRECTION ( 'NONE',  ( 0.1728608224830406603, 1.098208118798718614E-16, -0.9849462604886047856 ) ) ;
#15162=DIRECTION ( 'NONE',  ( 9.627370216492862708E-17, 1.000000000000000000, -0.000000000000000000 ) ) ;
#15180=EDGE_CURVE ( 'NONE', #18529, #41231, #8629, .T. ) ;
#15186=ORIENTED_EDGE ( 'NONE', *, *, #36531, .F. ) ;
#15194=AXIS2_PLACEMENT_3D ( 'NONE', #24950, #23518, #24154 ) ;
#15208=B_SPLINE_CURVE_WITH_KNOTS ( 'NONE', 3,
 ( #28795, #38802, #31782, #2827 ),
 .UNSPECIFIED., .F., .F.,
 ( 4, 4 ),
 ( 0.02831029896240152416, 1.000000000000000000 ),
 .UNSPECIFIED. ) ;
#15209=( BOUNDED_CURVE ( )  B_SPLINE_CURVE ( 3, ( #14675, #28311, #40691, #18707 ),
 .UNSPECIFIED., .F., .T. ) 
 B_SPLINE_CURVE_WITH_KNOTS ( ( 4, 4 ),
 ( 0.6093138467282536164, 1.570796326794897002 ),
 .UNSPECIFIED. ) 
 CURVE ( )  GEOMETRIC_REPRESENTATION_ITEM ( )  RATIONAL_B_SPLINE_CURVE ( ( 1.000000000000000000, 0.9244349266169026302, 0.9244349266169026302, 1.000000000000000000 ) ) 
 REPRESENTATION_ITEM ( '' )  );
#15210=CARTESIAN_POINT ( 'NONE',  ( 1.248107678658480997E-15, 12.96416000000000146, 0.000000000000000000 ) ) ;
#15219=ORIENTED_EDGE ( 'NONE', *, *, #3029, .T. ) ;
#15222=DIRECTION ( 'NONE',  ( -0.000000000000000000, 1.000000000000000000, 0.000000000000000000 ) ) ;
#15234=CARTESIAN_POINT ( 'NONE',  ( 17.14499999999999957, 71.11999999999999034, 1.904999999999989146 ) ) ;
#15238=CARTESIAN_POINT ( 'NONE',  ( -10.28897677580358305, 57.14999999999998437, 4.381499999999999950 ) ) ;
#15239=VERTEX_POINT ( 'NONE', #27173 ) ;
#15251=CARTESIAN_POINT ( 'NONE',  ( -12.87096146653068196, 58.93153423982063543, -10.60403923708992835 ) ) ;
#15252=CARTESIAN_POINT ( 'NONE',  ( 4.968814169093906941, 56.51947256399660802, 4.801687862347802316 ) ) ;
#15262=CARTESIAN_POINT ( 'NONE',  ( 5.322311913656744942, 57.14999999999977831, -5.239113282063458499 ) ) ;
#15272=CARTESIAN_POINT ( 'NONE',  ( -10.19284229789036900, 16.51000000000000156, 4.908176479697702099 ) ) ;
#15304=EDGE_LOOP ( 'NONE', ( #9423, #15089, #6568, #18157 ) ) ;
#15311=CARTESIAN_POINT ( 'NONE',  ( 12.69999999999999929, 14.60500000000000043, 1.555301434917138235E-15 ) ) ;
#15312=CARTESIAN_POINT ( 'NONE',  ( -10.96186877710140273, 56.39406130473899736, 5.016500000001508752 ) ) ;
#15317=VERTEX_POINT ( 'NONE', #40390 ) ;
#15323=CARTESIAN_POINT ( 'NONE',  ( -13.85159022459153988, 12.96416000000000146, 5.016499999999999737 ) ) ;
#15327=DIRECTION ( 'NONE',  ( 1.000000000000000000, 0.000000000000000000, 1.224646799147354933E-16 ) ) ;
#15338=ORIENTED_EDGE ( 'NONE', *, *, #42104, .F. ) ;
#15358=ORIENTED_EDGE ( 'NONE', *, *, #15764, .T. ) ;
#15361=PLANE ( 'NONE',  #2819 ) ;
#15368=EDGE_CURVE ( 'NONE', #15239, #9633, #17237, .T. ) ;
#15386=ORIENTED_EDGE ( 'NONE', *, *, #37572, .F. ) ;
#15412=EDGE_CURVE ( 'NONE', #29525, #18747, #12471, .T. ) ;
#15416=DIRECTION ( 'NONE',  ( 1.000000000000000000, 0.000000000000000000, -6.146657985744592735E-16 ) ) ;
#15428=LINE ( 'NONE', #8418, #1161 ) ;
#15429=CARTESIAN_POINT ( 'NONE',  ( -5.965356522962928842, 65.30181249999998272, -5.016499999999999737 ) ) ;
#15443=AXIS2_PLACEMENT_3D ( 'NONE', #21759, #18575, #4987 ) ;
#15467=ORIENTED_EDGE ( 'NONE', *, *, #2134, .F. ) ;
#15471=CARTESIAN_POINT ( 'NONE',  ( -16.60960244842765832, 1.599067919197793490E-15, 0.000000000000000000 ) ) ;
#15483=LINE ( 'NONE', #16477, #14370 ) ;
#15497=DIRECTION ( 'NONE',  ( 1.000000000000000000, -1.365923996832131856E-16, 0.000000000000000000 ) ) ;
#15508=ORIENTED_EDGE ( 'NONE', *, *, #29812, .T. ) ;
#15518=EDGE_LOOP ( 'NONE', ( #24301, #19186, #20768, #24676, #21892, #39585, #3906, #21283, #22534, #5466, #29652, #25812 ) ) ;
#15522=EDGE_CURVE ( 'NONE', #16450, #10948, #28794, .T. ) ;
#15526=CARTESIAN_POINT ( 'NONE',  ( -11.25890006629609097, 56.90956307411621395, 5.016499999999999737 ) ) ;
#15527=DIRECTION ( 'NONE',  ( 1.000000000000000000, -9.627370216492862708E-17, 0.000000000000000000 ) ) ;
#15530=CARTESIAN_POINT ( 'NONE',  ( -7.213960532363670630, 78.77618639008812806, 1.904999999999999583 ) ) ;
#15532=EDGE_LOOP ( 'NONE', ( #7622, #493, #5343, #31007, #9589, #33068 ) ) ;
#15551=ORIENTED_EDGE ( 'NONE', *, *, #4596, .F. ) ;
#15557=EDGE_LOOP ( 'NONE', ( #39856, #8552, #3426, #3652, #11469, #1892 ) ) ;
#15559=CARTESIAN_POINT ( 'NONE',  ( -14.73199999999999577, 61.59499999999999886, 1.904999999999990479 ) ) ;
#15578=FACE_OUTER_BOUND ( 'NONE', #1121, .T. ) ;
#15581=LINE ( 'NONE', #3036, #24379 ) ;
#15590=FACE_OUTER_BOUND ( 'NONE', #18223, .T. ) ;
#15595=CARTESIAN_POINT ( 'NONE',  ( 6.059261036834406866, 65.30181249999998272, 5.016499999999999737 ) ) ;
#15597=VERTEX_POINT ( 'NONE', #9773 ) ;
#15619=CARTESIAN_POINT ( 'NONE',  ( -11.58677707360137532, 55.24499999999999034, -4.474811398758259173 ) ) ;
#15622=PLANE ( 'NONE',  #38953 ) ;
#15623=AXIS2_PLACEMENT_3D ( 'NONE', #15238, #18642, #41031 ) ;
#15626=LINE ( 'NONE', #38650, #32401 ) ;
#15634=CARTESIAN_POINT ( 'NONE',  ( -5.871452009091383317, 53.58606249999999704, -5.016499999999999737 ) ) ;
#15651=EDGE_CURVE ( 'NONE', #14687, #4530, #4055, .T. ) ;
#15654=DIRECTION ( 'NONE',  ( 0.000000000000000000, 0.000000000000000000, 1.000000000000000000 ) ) ;
#15668=ADVANCED_FACE ( 'NONE', ( #32355, #3183 ), #207, .T. ) ;
#15674=CARTESIAN_POINT ( 'NONE',  ( -4.792324638262678960, 56.51998046905272588, 4.972049999962470324 ) ) ;
#15682=DIRECTION ( 'NONE',  ( -9.627370216492862708E-17, -1.000000000000000000, 0.000000000000000000 ) ) ;
#15684=CARTESIAN_POINT ( 'NONE',  ( -5.936145915410568463, 56.51499999999997925, 4.381499802576774627 ) ) ;
#15686=ORIENTED_EDGE ( 'NONE', *, *, #11633, .F. ) ;
#15695=ADVANCED_FACE ( 'NONE', ( #1264 ), #7063, .T. ) ;
#15697=CARTESIAN_POINT ( 'NONE',  ( 7.213960532363571154, 78.77618639008812806, -1.904999999999999583 ) ) ;
#15699=DIRECTION ( 'NONE',  ( -9.627370216492862708E-17, -1.000000000000000000, 0.000000000000000000 ) ) ;
#15704=CARTESIAN_POINT ( 'NONE',  ( 5.224085778414913506, 56.51499999999996504, 4.542437760755090537 ) ) ;
#15711=EDGE_LOOP ( 'NONE', ( #4416, #37911, #3185, #12781, #40616, #18643 ) ) ;
#15721=DIRECTION ( 'NONE',  ( 1.000000000000000000, 0.000000000000000000, -6.146657985744586818E-16 ) ) ;
#15722=VECTOR ( 'NONE', #37312, 1000.000000000000000 ) ;
#15732=DIRECTION ( 'NONE',  ( -0.9849462604886047856, 0.000000000000000000, 0.1728608224830407714 ) ) ;
#15742=FACE_OUTER_BOUND ( 'NONE', #28509, .T. ) ;
#15764=EDGE_CURVE ( 'NONE', #13560, #24559, #31249, .T. ) ;
#15803=CARTESIAN_POINT ( 'NONE',  ( 5.871452009091314039, 65.30181249999998272, 5.016499999999999737 ) ) ;
#15810=EDGE_CURVE ( 'NONE', #16922, #329, #24045, .T. ) ;
#15816=LINE ( 'NONE', #9028, #1907 ) ;
#15821=CARTESIAN_POINT ( 'NONE',  ( -6.262914499211170494, 78.85772796343783853, 4.069400916056300943 ) ) ;
#15830=CARTESIAN_POINT ( 'NONE',  ( 9.094996104468805243, 78.64197151092925253, -1.904999999999999583 ) ) ;
#15839=EDGE_LOOP ( 'NONE', ( #32024, #18230, #11513, #15686 ) ) ;
#15852=ORIENTED_EDGE ( 'NONE', *, *, #16581, .F. ) ;
#15861=CARTESIAN_POINT ( 'NONE',  ( -5.177913976931285411, 57.14999999999998437, 5.372100000000002318 ) ) ;
#15866=VERTEX_POINT ( 'NONE', #26743 ) ;
#15886=VECTOR ( 'NONE', #32437, 1000.000000000000000 ) ;
#15899=AXIS2_PLACEMENT_3D ( 'NONE', #14812, #34852, #15654 ) ;
#15903=EDGE_CURVE ( 'NONE', #25560, #26298, #41730, .T. ) ;
#15904=ORIENTED_EDGE ( 'NONE', *, *, #18547, .F. ) ;
#15919=VERTEX_POINT ( 'NONE', #7985 ) ;
#15929=CARTESIAN_POINT ( 'NONE',  ( 5.106395947886047004, 78.95054594174945350, 5.392902600000138769 ) ) ;
#15938=CARTESIAN_POINT ( 'NONE',  ( 5.614623559985534307, 78.91041036408813625, 5.070733448224204132 ) ) ;
#15959=CARTESIAN_POINT ( 'NONE',  ( 6.059261036834405090, 56.51500000000000057, -4.381499999999999950 ) ) ;
#15962=EDGE_LOOP ( 'NONE', ( #18435, #40701, #13473, #3074, #41227, #9396, #36780, #4840 ) ) ;
#16010=ORIENTED_EDGE ( 'NONE', *, *, #9209, .F. ) ;
#16041=ADVANCED_FACE ( 'NONE', ( #11222 ), #9757, .T. ) ;
#16051=CARTESIAN_POINT ( 'NONE',  ( 6.059261036833980540, 78.87450423423040036, -5.016499999999999737 ) ) ;
#16056=ORIENTED_EDGE ( 'NONE', *, *, #2384, .F. ) ;
#16073=ORIENTED_EDGE ( 'NONE', *, *, #27913, .F. ) ;
#16085=DIRECTION ( 'NONE',  ( 9.627370216492862708E-17, 1.000000000000000000, -0.000000000000000000 ) ) ;
#16099=AXIS2_PLACEMENT_3D ( 'NONE', #9010, #5619, #34160 ) ;
#16107=CARTESIAN_POINT ( 'NONE',  ( 6.059261036834405090, 56.51500000000000057, -4.381499999999999950 ) ) ;
#16120=CARTESIAN_POINT ( 'NONE',  ( 5.354045385558688253, 56.51499999999995794, 5.213862164400304700 ) ) ;
#16132=CARTESIAN_POINT ( 'NONE',  ( -1.925929944387235853E-31, 0.000000000000000000, 0.000000000000000000 ) ) ;
#16136=CARTESIAN_POINT ( 'NONE',  ( 11.66725022231030984, 17.14499999999999957, 5.016499999999999737 ) ) ;
#16139=CARTESIAN_POINT ( 'NONE',  ( -5.449227423778994606, 57.14999999999997726, -5.145694933688813144 ) ) ;
#16141=CARTESIAN_POINT ( 'NONE',  ( 5.675123159882344837, 78.90545016724973948, 5.052246757648558351 ) ) ;
#16146=CARTESIAN_POINT ( 'NONE',  ( -5.981046608238790974, 78.88093534801386397, -5.016500000000000625 ) ) ;
#16155=CYLINDRICAL_SURFACE ( 'NONE', #922, 1.270000000000000240 ) ;
#16156=CARTESIAN_POINT ( 'NONE',  ( 12.69999999999999929, 16.51000000000000156, 1.555301434917138235E-15 ) ) ;
#16172=B_SPLINE_CURVE_WITH_KNOTS ( 'NONE', 3,
 ( #609, #19146, #12759, #22323 ),
 .UNSPECIFIED., .F., .F.,
 ( 4, 4 ),
 ( 0.000000000000000000, 0.9716897010375996624 ),
 .UNSPECIFIED. ) ;
#16175=ORIENTED_EDGE ( 'NONE', *, *, #19746, .T. ) ;
#16192=B_SPLINE_CURVE_WITH_KNOTS ( 'NONE', 3,
 ( #21147, #20945, #14556, #33970, #27563, #24356 ),
 .UNSPECIFIED., .F., .F.,
 ( 4, 2, 4 ),
 ( 0.000000000000000000, 0.5000000000000000000, 1.000000000000000000 ),
 .UNSPECIFIED. ) ;
#16193=DIRECTION ( 'NONE',  ( 0.000000000000000000, 1.000000000000000000, 0.000000000000000000 ) ) ;
#16206=VECTOR ( 'NONE', #19202, 1000.000000000000000 ) ;
#16210=CARTESIAN_POINT ( 'NONE',  ( 1.650612623617701257E-15, 17.14499999999999957, 0.000000000000000000 ) ) ;
#16216=EDGE_CURVE ( 'NONE', #36071, #13136, #10140, .T. ) ;
#16228=CARTESIAN_POINT ( 'NONE',  ( -6.350000000000036060, 57.14999999999998437, 7.776507174585692163E-16 ) ) ;
#16240=ORIENTED_EDGE ( 'NONE', *, *, #914, .T. ) ;
#16248=CARTESIAN_POINT ( 'NONE',  ( -13.85159022459153988, 12.96416000000000146, -5.016499999999999737 ) ) ;
#16264=EDGE_CURVE ( 'NONE', #18747, #6508, #19266, .T. ) ;
#16271=ORIENTED_EDGE ( 'NONE', *, *, #6873, .T. ) ;
#16272=CARTESIAN_POINT ( 'NONE',  ( 16.87828382557106721, 4.021169087505850551E-17, 0.000000000000000000 ) ) ;
#16287=EDGE_LOOP ( 'NONE', ( #21343, #31078, #26364, #7018 ) ) ;
#16301=ORIENTED_EDGE ( 'NONE', *, *, #2888, .F. ) ;
#16309=LINE ( 'NONE', #29095, #19515 ) ;
#16317=UNCERTAINTY_MEASURE_WITH_UNIT (LENGTH_MEASURE( 1.000000000000000082E-05 ), #37942, 'distance_accuracy_value', 'NONE');
#16330=CARTESIAN_POINT ( 'NONE',  ( 17.14499999999999957, 71.11999999999999034, 5.016499999999999737 ) ) ;
#16336=CARTESIAN_POINT ( 'NONE',  ( 4.918266948218991352, 56.51499999999997215, 4.748921713023384505 ) ) ;
#16344=VECTOR ( 'NONE', #23421, 1000.000000000000000 ) ;
#16347=ORIENTED_EDGE ( 'NONE', *, *, #6404, .F. ) ;
#16349=DIRECTION ( 'NONE',  ( 9.627370216492862708E-17, 1.000000000000000000, -0.000000000000000000 ) ) ;
#16352=AXIS2_PLACEMENT_3D ( 'NONE', #13547, #1404, #6955 ) ;
#16354=CARTESIAN_POINT ( 'NONE',  ( -13.85159022459154166, 60.48513866567135722, 5.016500000000000625 ) ) ;
#16358=DIRECTION ( 'NONE',  ( 0.000000000000000000, -0.000000000000000000, 1.000000000000000000 ) ) ;
#16362=CARTESIAN_POINT ( 'NONE',  ( -5.624629865489270131, 78.90958242041959636, -5.067363953418781541 ) ) ;
#16368=AXIS2_PLACEMENT_3D ( 'NONE', #37902, #18083, #15721 ) ;
#16373=CARTESIAN_POINT ( 'NONE',  ( 1.650612623617701257E-15, 17.14499999999999957, 0.000000000000000000 ) ) ;
#16377=CARTESIAN_POINT ( 'NONE',  ( -13.76130258807007500, 16.83823567964705958, -5.016499999999998849 ) ) ;
#16383=ORIENTED_EDGE ( 'NONE', *, *, #3424, .T. ) ;
#16390=ORIENTED_EDGE ( 'NONE', *, *, #17820, .T. ) ;
#16403=ORIENTED_EDGE ( 'NONE', *, *, #7939, .T. ) ;
#16404=DIRECTION ( 'NONE',  ( -1.000000000000000000, 0.000000000000000000, 0.000000000000000000 ) ) ;
#16408=CARTESIAN_POINT ( 'NONE',  ( -13.83234216238653680, 16.68269501491596785, 5.016499999999998849 ) ) ;
#16421=CIRCLE ( 'NONE', #37533, 2.540000000000000480 ) ;
#16427=CARTESIAN_POINT ( 'NONE',  ( 11.66725022231030984, 16.51000000000000156, -5.016499999999999737 ) ) ;
#16439=EDGE_CURVE ( 'NONE', #11659, #4497, #28623, .T. ) ;
#16446=CARTESIAN_POINT ( 'NONE',  ( 13.17422243436029916, 17.14500000000093394, -5.016499999999999737 ) ) ;
#16450=VERTEX_POINT ( 'NONE', #15619 ) ;
#16452=EDGE_CURVE ( 'NONE', #41795, #34762, #30161, .T. ) ;
#16454=ORIENTED_EDGE ( 'NONE', *, *, #9224, .F. ) ;
#16465=DIRECTION ( 'NONE',  ( -0.000000000000000000, -0.000000000000000000, -1.000000000000000000 ) ) ;
#16466=ADVANCED_FACE ( 'NONE', ( #22208 ), #22820, .F. ) ;
#16468=ADVANCED_FACE ( 'NONE', ( #3499 ), #29466, .T. ) ;
#16477=CARTESIAN_POINT ( 'NONE',  ( -14.73199999999999754, 61.59499999999999886, -1.904999999999999583 ) ) ;
#16482=ORIENTED_EDGE ( 'NONE', *, *, #20903, .F. ) ;
#16493=DIRECTION ( 'NONE',  ( 1.000000000000000000, 0.000000000000000000, 0.000000000000000000 ) ) ;
#16503=DIRECTION ( 'NONE',  ( 6.353134868986659519E-16, -1.000000000000000000, 0.000000000000000000 ) ) ;
#16510=VECTOR ( 'NONE', #5860, 1000.000000000000000 ) ;
#16516=DIRECTION ( 'NONE',  ( 0.000000000000000000, 0.000000000000000000, -1.000000000000000000 ) ) ;
#16522=DIRECTION ( 'NONE',  ( 0.000000000000000000, 1.000000000000000000, 0.000000000000000000 ) ) ;
#16531=EDGE_CURVE ( 'NONE', #40888, #21156, #23782, .T. ) ;
#16533=EDGE_LOOP ( 'NONE', ( #14583, #8179, #28768, #31770 ) ) ;
#16540=CARTESIAN_POINT ( 'NONE',  ( 14.95453923199683111, 61.75387968257833649, 5.016499999999999737 ) ) ;
#16545=CARTESIAN_POINT ( 'NONE',  ( -14.95453923199683288, 61.75387968257833649, -5.016499999999999737 ) ) ;
#16546=CARTESIAN_POINT ( 'NONE',  ( -1.925929944387235853E-31, 0.000000000000000000, 0.000000000000000000 ) ) ;
#16553=VECTOR ( 'NONE', #36722, 1000.000000000000114 ) ;
#16556=ORIENTED_EDGE ( 'NONE', *, *, #12782, .T. ) ;
#16557=VECTOR ( 'NONE', #28467, 1000.000000000000000 ) ;
#16577=CARTESIAN_POINT ( 'NONE',  ( -17.14499999999999957, 71.11999999999999034, 5.016499999999999737 ) ) ;
#16581=EDGE_CURVE ( 'NONE', #11659, #28739, #38900, .T. ) ;
#16582=( BOUNDED_CURVE ( )  B_SPLINE_CURVE ( 3, ( #25737, #35554, #29788, #26586 ),
 .UNSPECIFIED., .F., .T. ) 
 B_SPLINE_CURVE_WITH_KNOTS ( ( 4, 4 ),
 ( 3.141592653589792672, 4.712388980384688786 ),
 .UNSPECIFIED. ) 
 CURVE ( )  GEOMETRIC_REPRESENTATION_ITEM ( )  RATIONAL_B_SPLINE_CURVE ( ( 1.000000000000000000, 0.8047378541243650485, 0.8047378541243650485, 1.000000000000000000 ) ) 
 REPRESENTATION_ITEM ( '' )  );
#16598=CARTESIAN_POINT ( 'NONE',  ( 1.332716859069107315E-15, 13.84300000000000352, 0.000000000000000000 ) ) ;
#16605=ORIENTED_EDGE ( 'NONE', *, *, #18079, .F. ) ;
#16621=DIRECTION ( 'NONE',  ( 0.000000000000000000, 0.000000000000000000, 1.000000000000000000 ) ) ;
#16622=DIRECTION ( 'NONE',  ( 0.000000000000000000, 1.000000000000000000, 0.000000000000000000 ) ) ;
#16627=LINE ( 'NONE', #17049, #41937 ) ;
#16635=DIRECTION ( 'NONE',  ( -0.000000000000000000, -0.000000000000000000, -1.000000000000000000 ) ) ;
#16646=VERTEX_POINT ( 'NONE', #6840 ) ;
#16668=EDGE_CURVE ( 'NONE', #37437, #37954, #28038, .T. ) ;
#16680=CARTESIAN_POINT ( 'NONE',  ( 6.758480964575337424, 78.81581826900307419, 3.179117336685197248 ) ) ;
#16682=CARTESIAN_POINT ( 'NONE',  ( 11.58677707360137710, 55.24500000000000455, -4.474811398758258285 ) ) ;
#16685=FACE_OUTER_BOUND ( 'NONE', #6319, .T. ) ;
#16689=EDGE_CURVE ( 'NONE', #13136, #19376, #7618, .T. ) ;
#16705=CARTESIAN_POINT ( 'NONE',  ( 5.241362157049057835, 57.14999999999999858, -5.310945289804168468 ) ) ;
#16706=DIRECTION ( 'NONE',  ( -0.5810519254489896479, 0.8138664877804110409, 0.000000000000000000 ) ) ;
#16740=EDGE_LOOP ( 'NONE', ( #34894, #35185, #33492, #27714 ) ) ;
#16744=ORIENTED_EDGE ( 'NONE', *, *, #4875, .F. ) ;
#16750=CARTESIAN_POINT ( 'NONE',  ( -6.266702236064261911, 78.85741254032745928, -4.063604302808976776 ) ) ;
#16752=VERTEX_POINT ( 'NONE', #13856 ) ;
#16769=VECTOR ( 'NONE', #38956, 1000.000000000000000 ) ;
#16778=CARTESIAN_POINT ( 'NONE',  ( -14.50851225146815437, 78.09971119798315442, 1.904999999999988258 ) ) ;
#16786=CARTESIAN_POINT ( 'NONE',  ( -5.511339492711898380, 56.51500000000000767, -5.111277471823950869 ) ) ;
#16794=CARTESIAN_POINT ( 'NONE',  ( -12.21488373879589240, 55.24499999999999034, -4.381499999999999950 ) ) ;
#16837=DIRECTION ( 'NONE',  ( -0.000000000000000000, -0.000000000000000000, -1.000000000000000000 ) ) ;
#16839=( BOUNDED_SURFACE ( )  B_SPLINE_SURFACE ( 3, 2, ( 
 ( #8350, #30295, #4964 ),
 ( #36915, #33932, #11123 ),
 ( #21320, #10909, #24111 ),
 ( #17713, #4761, #34348 ),
 ( #20484, #26894, #7733 ),
 ( #23899, #932, #30712 ),
 ( #30506, #37119, #37527 ),
 ( #5179, #18132, #33510 ),
 ( #27530, #1561, #21113 ),
 ( #4344, #13904, #17306 ) ),
 .UNSPECIFIED., .F., .F., .F. ) 
 B_SPLINE_SURFACE_WITH_KNOTS ( ( 4, 2, 2, 2, 4 ),
 ( 3, 3 ),
 ( 3.141592653589792672, 3.534291735288516811, 3.926990816987241395, 4.319689898685965090, 4.712388980384689674 ),
 ( 0.000000000000000000, 1.000000000000000000 ),
 .UNSPECIFIED. ) 
 GEOMETRIC_REPRESENTATION_ITEM ( )  RATIONAL_B_SPLINE_SURFACE ( (
 ( 1.000000000000000000, 0.7572803591334824613, 1.000000000000000000),
 ( 1.000000000000000000, 0.7572851909592176467, 1.000000000000000000),
 ( 1.000000000000000000, 0.7560206254140762194, 1.000000000000000000),
 ( 1.000000000000000000, 0.7511365686956508192, 1.000000000000000000),
 ( 1.000000000000000000, 0.7475127447244064305, 1.000000000000000000),
 ( 1.000000000000000000, 0.7383589052088851412, 1.000000000000000000),
 ( 1.000000000000000000, 0.7328301610707728120, 1.000000000000000000),
 ( 1.000000000000000000, 0.7206031636698049248, 1.000000000000000000),
 ( 1.000000000000000000, 0.7139102541742058383, 1.000000000000000000),
 ( 1.000000000000000000, 0.7071067811865475727, 1.000000000000000000) ) ) 
 REPRESENTATION_ITEM ( '' )  SURFACE ( )  );
#16850=CARTESIAN_POINT ( 'NONE',  ( -5.809014734623222154, 78.89492211486511053, 5.027281507146216910 ) ) ;
#16854=DIRECTION ( 'NONE',  ( -1.000000000000000000, 9.627370216492862708E-17, 0.000000000000000000 ) ) ;
#16862=ORIENTED_EDGE ( 'NONE', *, *, #20903, .T. ) ;
#16897=B_SPLINE_CURVE_WITH_KNOTS ( 'NONE', 3,
 ( #7351, #17340, #26514, #33336 ),
 .UNSPECIFIED., .F., .F.,
 ( 4, 4 ),
 ( 0.000000000000000000, 0.5094958736258423659 ),
 .UNSPECIFIED. ) ;
#16909=DIRECTION ( 'NONE',  ( -9.627370216492862708E-17, -1.000000000000000000, 0.000000000000000000 ) ) ;
#16922=VERTEX_POINT ( 'NONE', #17260 ) ;
#16941=LINE ( 'NONE', #23526, #2088 ) ;
#16964=CARTESIAN_POINT ( 'NONE',  ( -6.059261036834082681, 78.87450423423038615, 5.016499999999999737 ) ) ;
#16975=ADVANCED_FACE ( 'NONE', ( #14262 ), #36239, .T. ) ;
#16981=EDGE_CURVE ( 'NONE', #24940, #32109, #10026, .T. ) ;
#16982=ORIENTED_EDGE ( 'NONE', *, *, #31827, .T. ) ;
#16993=DIRECTION ( 'NONE',  ( -0.1728608224830406603, 0.000000000000000000, -0.9849462604886047856 ) ) ;
#17039=VERTEX_POINT ( 'NONE', #4713 ) ;
#17040=FACE_OUTER_BOUND ( 'NONE', #30924, .T. ) ;
#17049=CARTESIAN_POINT ( 'NONE',  ( -23.49500000000000455, 71.11999999999999034, 5.016499999999999737 ) ) ;
#17056=CARTESIAN_POINT ( 'NONE',  ( -5.692269266618634305, 78.90431106374057890, 5.047924920909140134 ) ) ;
#17081=DIRECTION ( 'NONE',  ( 1.000000000000000000, 0.000000000000000000, 0.000000000000000000 ) ) ;
#17095=CIRCLE ( 'NONE', #32076, 0.6350000000000001199 ) ;
#17103=AXIS2_PLACEMENT_3D ( 'NONE', #34658, #18873, #37424 ) ;
#17109=CARTESIAN_POINT ( 'NONE',  ( 1.247998466936323035E-15, 12.96302561210691806, 0.000000000000000000 ) ) ;
#17112=CARTESIAN_POINT ( 'NONE',  ( 14.73199999999999932, 12.96416000000000146, 0.000000000000000000 ) ) ;
#17114=VERTEX_POINT ( 'NONE', #16136 ) ;
#17121=AXIS2_PLACEMENT_3D ( 'NONE', #27547, #24337, #34158 ) ;
#17129=CARTESIAN_POINT ( 'NONE',  ( 5.177913976931212581, 57.15000000000004832, -5.372100000000001430 ) ) ;
#17177=CARTESIAN_POINT ( 'NONE',  ( -6.059261036834486802, 71.63300248836199557, 5.016499999999999737 ) ) ;
#17178=DIRECTION ( 'NONE',  ( 0.9891443546370349837, 0.000000000000000000, -0.1469470846586742874 ) ) ;
#17179=EDGE_LOOP ( 'NONE', ( #22662, #41671, #14645, #16175, #23620, #7986, #39041, #26256, #13352, #6751, #42050, #41305 ) ) ;
#17188=ORIENTED_EDGE ( 'NONE', *, *, #15412, .T. ) ;
#17189=B_SPLINE_CURVE_WITH_KNOTS ( 'NONE', 3,
 ( #24906, #41325, #5135, #21690 ),
 .UNSPECIFIED., .F., .F.,
 ( 4, 4 ),
 ( 0.02839955696672210456, 1.000000000000000000 ),
 .UNSPECIFIED. ) ;
#17196=LINE ( 'NONE', #7837, #18913 ) ;
#17199=AXIS2_PLACEMENT_3D ( 'NONE', #11234, #23586, #16993 ) ;
#17206=FACE_OUTER_BOUND ( 'NONE', #6286, .T. ) ;
#17237=CIRCLE ( 'NONE', #26082, 14.73199999999999577 ) ;
#17239=ORIENTED_EDGE ( 'NONE', *, *, #20088, .F. ) ;
#17254=ORIENTED_EDGE ( 'NONE', *, *, #11201, .T. ) ;
#17260=CARTESIAN_POINT ( 'NONE',  ( -18.32410244842765934, 0.6350000000000018963, 0.000000000000000000 ) ) ;
#17262=CARTESIAN_POINT ( 'NONE',  ( 1.650612623617701454E-15, 17.14499999999999957, 0.000000000000000000 ) ) ;
#17265=CARTESIAN_POINT ( 'NONE',  ( -17.14499999999999957, 71.11999999999999034, -5.016499999999999737 ) ) ;
#17273=AXIS2_PLACEMENT_3D ( 'NONE', #19330, #25727, #3377 ) ;
#17278=CARTESIAN_POINT ( 'NONE',  ( 1.589478822742971486E-15, 16.51000000000000156, 0.000000000000000000 ) ) ;
#17302=EDGE_LOOP ( 'NONE', ( #32219, #36368, #12758, #25365 ) ) ;
#17303=B_SPLINE_CURVE_WITH_KNOTS ( 'NONE', 3,
 ( #8240, #8036, #24843, #31230, #21211, #21009 ),
 .UNSPECIFIED., .F., .F.,
 ( 4, 2, 4 ),
 ( 0.0008205648557148674267, 0.001333860798246176271, 0.001847156740777485115 ),
 .UNSPECIFIED. ) ;
#17306=CARTESIAN_POINT ( 'NONE',  ( 10.28897677580358128, 57.14999999999999858, -5.016500000000000625 ) ) ;
#17318=DIRECTION ( 'NONE',  ( -0.7071067811865467956, -0.7071067811865483499, 8.659560562354924230E-17 ) ) ;
#17331=DIRECTION ( 'NONE',  ( 6.353134868986659519E-16, -1.000000000000000000, 0.000000000000000000 ) ) ;
#17340=CARTESIAN_POINT ( 'NONE',  ( -15.15189561879878433, 77.97492127061543954, -1.904999999999999583 ) ) ;
#17378=ORIENTED_EDGE ( 'NONE', *, *, #86, .F. ) ;
#17385=EDGE_LOOP ( 'NONE', ( #19918, #6796 ) ) ;
#17388=CARTESIAN_POINT ( 'NONE',  ( 13.85159022459153988, 16.51000000000000156, 5.016499999999999737 ) ) ;
#17389=DIRECTION ( 'NONE',  ( 1.000000000000000000, 0.000000000000000000, -0.000000000000000000 ) ) ;
#17420=VERTEX_POINT ( 'NONE', #29246 ) ;
#17428=VECTOR ( 'NONE', #1485, 1000.000000000000000 ) ;
#17435=TOROIDAL_SURFACE ( 'NONE', #41263, 14.09699999999999420, 0.6350000000000000089 ) ;
#17438=CARTESIAN_POINT ( 'NONE',  ( 11.65115770210962687, 16.51000000000000156, 4.908176479697702099 ) ) ;
#17444=VERTEX_POINT ( 'NONE', #13274 ) ;
#17463=LINE ( 'NONE', #33884, #24550 ) ;
#17466=DIRECTION ( 'NONE',  ( -1.000000000000000000, 1.893378931774809890E-16, 0.000000000000000000 ) ) ;
#17468=CARTESIAN_POINT ( 'NONE',  ( 18.35410564743290607, 77.35382415001784295, 5.016499999999999737 ) ) ;
#17475=LINE ( 'NONE', #688, #12814 ) ;
#17481=CARTESIAN_POINT ( 'NONE',  ( -5.177913976931285411, 57.14999999999999858, -5.372100000000001430 ) ) ;
#17487=CIRCLE ( 'NONE', #22908, 7.461249999999999716 ) ;
#17505=EDGE_LOOP ( 'NONE', ( #22181, #33300, #21912, #8337, #3161, #36174, #35558, #7535 ) ) ;
#17526=DIRECTION ( 'NONE',  ( -0.5810519254489896479, -0.8138664877804110409, 0.000000000000000000 ) ) ;
#17540=EDGE_CURVE ( 'NONE', #35348, #16752, #36701, .T. ) ;
#17542=CARTESIAN_POINT ( 'NONE',  ( 14.73199999999999754, 61.59499999999999886, 5.016499999999999737 ) ) ;
#17555=ADVANCED_FACE ( 'NONE', ( #11332 ), #16839, .T. ) ;
#17557=ORIENTED_EDGE ( 'NONE', *, *, #931, .F. ) ;
#17575=ORIENTED_EDGE ( 'NONE', *, *, #18882, .F. ) ;
#17584=CARTESIAN_POINT ( 'NONE',  ( 10.92199999999999704, 57.78500000000000369, 5.016499999999999737 ) ) ;
#17592=ADVANCED_FACE ( 'NONE', ( #14304 ), #23140, .T. ) ;
#17601=ORIENTED_EDGE ( 'NONE', *, *, #41067, .F. ) ;
#17611=DIRECTION ( 'NONE',  ( 6.146657985744592735E-16, 3.905054717696927382E-31, 1.000000000000000000 ) ) ;
#17616=DIRECTION ( 'NONE',  ( -0.1715592850456333085, 0.1224830539174543292, 0.9775302108976914317 ) ) ;
#17621=B_SPLINE_CURVE_WITH_KNOTS ( 'NONE', 3,
 ( #31038, #37650, #8475, #34666 ),
 .UNSPECIFIED., .F., .F.,
 ( 4, 4 ),
 ( 0.02831029896240370991, 1.000000000000000000 ),
 .UNSPECIFIED. ) ;
#17640=CARTESIAN_POINT ( 'NONE',  ( 13.46199999999999619, 17.14499999999999957, 1.648619521012166171E-15 ) ) ;
#17666=AXIS2_PLACEMENT_3D ( 'NONE', #17800, #4217, #17178 ) ;
#17667=LINE ( 'NONE', #24269, #27939 ) ;
#17680=CARTESIAN_POINT ( 'NONE',  ( -13.73816324777078890, 59.55066437026322745, 5.662797264199856073 ) ) ;
#17696=ORIENTED_EDGE ( 'NONE', *, *, #25329, .T. ) ;
#17701=CYLINDRICAL_SURFACE ( 'NONE', #23195, 2.539999999999999591 ) ;
#17710=ORIENTED_EDGE ( 'NONE', *, *, #2757, .T. ) ;
#17713=CARTESIAN_POINT ( 'NONE',  ( 11.42297701379735742, 55.88459609804034756, -4.463034230327253660 ) ) ;
#17730=CARTESIAN_POINT ( 'NONE',  ( -4.825814575782359839, 56.51500000000000767, 4.829586058641171853 ) ) ;
#17740=AXIS2_PLACEMENT_3D ( 'NONE', #8783, #34986, #18554 ) ;
#17771=ADVANCED_FACE ( 'NONE', ( #41798 ), #12596, .T. ) ;
#17783=DIRECTION ( 'NONE',  ( 0.000000000000000000, -0.000000000000000000, 1.000000000000000000 ) ) ;
#17784=ORIENTED_EDGE ( 'NONE', *, *, #33678, .T. ) ;
#17797=VECTOR ( 'NONE', #1699, 1000.000000000000114 ) ;
#17800=CARTESIAN_POINT ( 'NONE',  ( 10.39494437172059094, 55.24500000000000455, 5.094799277214218769 ) ) ;
#17801=ORIENTED_EDGE ( 'NONE', *, *, #6848, .F. ) ;
#17817=EDGE_LOOP ( 'NONE', ( #38199, #36391, #16454, #11750 ) ) ;
#17820=EDGE_CURVE ( 'NONE', #3641, #18200, #5599, .T. ) ;
#17824=ADVANCED_FACE ( 'NONE', ( #1976 ), #15000, .T. ) ;
#17827=CARTESIAN_POINT ( 'NONE',  ( -5.486567272856878414E-14, 86.35999999999998522, 0.000000000000000000 ) ) ;
#17830=ADVANCED_FACE ( 'NONE', ( #37957 ), #15361, .F. ) ;
#17835=DIRECTION ( 'NONE',  ( -6.353134868986659519E-16, 1.000000000000000000, 0.000000000000000000 ) ) ;
#17836=ORIENTED_EDGE ( 'NONE', *, *, #11013, .T. ) ;
#17853=CARTESIAN_POINT ( 'NONE',  ( 5.475330206976777525, 77.01756249999996840, -5.107412922131463695 ) ) ;
#17868=CIRCLE ( 'NONE', #22624, 0.6350000000000001199 ) ;
#17888=CARTESIAN_POINT ( 'NONE',  ( -23.49500000000000455, 71.11999999999999034, 5.016499999999999737 ) ) ;
#17913=DIRECTION ( 'NONE',  ( 0.1715592850456333085, 0.1224830539174543292, -0.9775302108976914317 ) ) ;
#17944=CARTESIAN_POINT ( 'NONE',  ( 1.650612623617701651E-15, 17.14499999999999957, 0.000000000000000000 ) ) ;
#17956=CIRCLE ( 'NONE', #10453, 0.6349999999999984546 ) ;
#17961=EDGE_LOOP ( 'NONE', ( #7678, #15551, #33368, #17801 ) ) ;
#17975=AXIS2_PLACEMENT_3D ( 'NONE', #32151, #25958, #12964 ) ;
#18005=EDGE_CURVE ( 'NONE', #25703, #1559, #32140, .T. ) ;
#18010=ORIENTED_EDGE ( 'NONE', *, *, #38619, .T. ) ;
#18019=VERTEX_POINT ( 'NONE', #22996 ) ;
#18023=CARTESIAN_POINT ( 'NONE',  ( 5.153327614265654333, 56.51694913689138389, 4.640534983550359094 ) ) ;
#18024=ORIENTED_EDGE ( 'NONE', *, *, #16216, .T. ) ;
#18037=CARTESIAN_POINT ( 'NONE',  ( -6.057513928997652286, 83.56599999999998829, 1.904999999999996030 ) ) ;
#18039=CARTESIAN_POINT ( 'NONE',  ( -3.630816577625875226E-14, 57.14999999999999147, 0.000000000000000000 ) ) ;
#18043=EDGE_CURVE ( 'NONE', #39961, #8736, #36449, .T. ) ;
#18046=DIRECTION ( 'NONE',  ( -0.000000000000000000, -0.000000000000000000, -1.000000000000000000 ) ) ;
#18057=EDGE_CURVE ( 'NONE', #10259, #3896, #3231, .T. ) ;
#18079=EDGE_CURVE ( 'NONE', #24559, #11189, #26212, .T. ) ;
#18083=DIRECTION ( 'NONE',  ( 6.146657985744592735E-16, 3.905054717696927382E-31, 1.000000000000000000 ) ) ;
#18086=CARTESIAN_POINT ( 'NONE',  ( -4.737240446979687825, 56.51500000000003610, -4.914900000000006486 ) ) ;
#18090=VECTOR ( 'NONE', #37917, 1000.000000000000114 ) ;
#18095=EDGE_LOOP ( 'NONE', ( #23085, #23569, #21695, #2803 ) ) ;
#18100=CARTESIAN_POINT ( 'NONE',  ( -11.97180806971932299, 56.20439414705996484, -5.016499999999999737 ) ) ;
#18118=VERTEX_POINT ( 'NONE', #26425 ) ;
#18122=DIRECTION ( 'NONE',  ( -1.000000000000000000, 0.000000000000000000, 0.000000000000000000 ) ) ;
#18132=CARTESIAN_POINT ( 'NONE',  ( 10.63219908769121247, 56.50600268266116188, -5.016500000000110759 ) ) ;
#18144=CIRCLE ( 'NONE', #35178, 0.6350000000000001199 ) ;
#18149=DIRECTION ( 'NONE',  ( 9.627370216492862708E-17, 1.000000000000000000, -0.000000000000000000 ) ) ;
#18155=ORIENTED_EDGE ( 'NONE', *, *, #38651, .T. ) ;
#18157=ORIENTED_EDGE ( 'NONE', *, *, #18596, .F. ) ;
#18174=AXIS2_PLACEMENT_3D ( 'NONE', #6579, #38748, #15527 ) ;
#18188=( BOUNDED_CURVE ( )  B_SPLINE_CURVE ( 3, ( #28805, #22383, #36043, #38812 ),
 .UNSPECIFIED., .F., .T. ) 
 B_SPLINE_CURVE_WITH_KNOTS ( ( 4, 4 ),
 ( 0.000000000000000000, 1.570796326794895226 ),
 .UNSPECIFIED. ) 
 CURVE ( )  GEOMETRIC_REPRESENTATION_ITEM ( )  RATIONAL_B_SPLINE_CURVE ( ( 1.000000000000000000, 0.8047378541243652705, 0.8047378541243652705, 1.000000000000000000 ) ) 
 REPRESENTATION_ITEM ( '' )  );
#18192=CIRCLE ( 'NONE', #42048, 16.60960244842765832 ) ;
#18200=VERTEX_POINT ( 'NONE', #9817 ) ;
#18213=EDGE_LOOP ( 'NONE', ( #14513, #20784, #19171, #8721, #17575 ) ) ;
#18223=EDGE_LOOP ( 'NONE', ( #2862, #28831, #17254, #22493, #30912, #31809, #26320, #36234, #16240, #13002, #34580, #24504 ) ) ;
#18230=ORIENTED_EDGE ( 'NONE', *, *, #12927, .T. ) ;
#18252=LINE ( 'NONE', #40657, #26754 ) ;
#18254=EDGE_CURVE ( 'NONE', #926, #15317, #6632, .T. ) ;
#18273=EDGE_LOOP ( 'NONE', ( #12593, #672, #8893, #20684 ) ) ;
#18279=EDGE_LOOP ( 'NONE', ( #32284, #1371 ) ) ;
#18284=EDGE_LOOP ( 'NONE', ( #37784, #7194 ) ) ;
#18287=DIRECTION ( 'NONE',  ( -0.000000000000000000, -0.000000000000000000, -1.000000000000000000 ) ) ;
#18296=CARTESIAN_POINT ( 'NONE',  ( 10.79307885933830136, 57.10041794475090171, 5.016499999999999737 ) ) ;
#18299=EDGE_LOOP ( 'NONE', ( #28599, #12539, #10799, #24463 ) ) ;
#18304=CARTESIAN_POINT ( 'NONE',  ( -11.62920297224728827, 55.59919541886078065, -5.016500000000107207 ) ) ;
#18330=DIRECTION ( 'NONE',  ( -1.224646799147353207E-16, -7.780346281855952181E-32, 1.000000000000000000 ) ) ;
#18334=DIRECTION ( 'NONE',  ( -1.000000000000000000, -1.092739197465705287E-15, 0.000000000000000000 ) ) ;
#18338=EDGE_CURVE ( 'NONE', #15239, #40888, #17463, .T. ) ;
#18339=ORIENTED_EDGE ( 'NONE', *, *, #40728, .T. ) ;
#18355=CYLINDRICAL_SURFACE ( 'NONE', #2215, 12.69999999999999751 ) ;
#18365=ORIENTED_EDGE ( 'NONE', *, *, #18254, .F. ) ;
#18417=DIRECTION ( 'NONE',  ( -9.627370216492862708E-17, -1.000000000000000000, 0.000000000000000000 ) ) ;
#18435=ORIENTED_EDGE ( 'NONE', *, *, #33633, .F. ) ;
#18446=CYLINDRICAL_SURFACE ( 'NONE', #17103, 14.73199999999999577 ) ;
#18450=DIRECTION ( 'NONE',  ( -0.9891443546370349837, 0.000000000000000000, -0.1469470846586743984 ) ) ;
#18453=CARTESIAN_POINT ( 'NONE',  ( 4.918180946948674581, 56.51499999999999346, -4.748993904426717982 ) ) ;
#18472=CARTESIAN_POINT ( 'NONE',  ( -12.21488373879589062, 56.36092316367925292, -5.016499999999999737 ) ) ;
#18490=AXIS2_PLACEMENT_3D ( 'NONE', #13458, #39448, #6440 ) ;
#18505=CARTESIAN_POINT ( 'NONE',  ( -3.590474171207809651E-14, 56.51499999999999346, 0.000000000000000000 ) ) ;
#18506=EDGE_CURVE ( 'NONE', #27187, #31705, #40221, .T. ) ;
#18509=VERTEX_POINT ( 'NONE', #27269 ) ;
#18510=DIRECTION ( 'NONE',  ( -0.000000000000000000, -0.000000000000000000, -1.000000000000000000 ) ) ;
#18514=CARTESIAN_POINT ( 'NONE',  ( -11.42297701379740893, 55.88459609804021255, -4.463034230327257212 ) ) ;
#18516=VECTOR ( 'NONE', #19155, 1000.000000000000114 ) ;
#18529=VERTEX_POINT ( 'NONE', #883 ) ;
#18536=ORIENTED_EDGE ( 'NONE', *, *, #7471, .F. ) ;
#18546=LINE ( 'NONE', #14721, #34496 ) ;
#18547=EDGE_CURVE ( 'NONE', #1374, #25364, #17667, .T. ) ;
#18553=DIRECTION ( 'NONE',  ( -0.1469470846586743706, -9.335746474409589170E-17, 0.9891443546370348727 ) ) ;
#18554=DIRECTION ( 'NONE',  ( 1.000000000000000000, -9.627370216492862708E-17, 0.000000000000000000 ) ) ;
#18565=EDGE_CURVE ( 'NONE', #1374, #30952, #23166, .T. ) ;
#18570=CARTESIAN_POINT ( 'NONE',  ( 11.58677707360137710, 55.24500000000000455, 4.474811398758258285 ) ) ;
#18575=DIRECTION ( 'NONE',  ( -0.000000000000000000, -0.000000000000000000, -1.000000000000000000 ) ) ;
#18581=ORIENTED_EDGE ( 'NONE', *, *, #16439, .T. ) ;
#18596=EDGE_CURVE ( 'NONE', #6334, #22648, #22105, .T. ) ;
#18614=DIRECTION ( 'NONE',  ( -0.000000000000000000, 0.000000000000000000, -1.000000000000000000 ) ) ;
#18622=CARTESIAN_POINT ( 'NONE',  ( -5.177913976931289852, 65.30181249999998272, -5.372100000000007647 ) ) ;
#18638=DIRECTION ( 'NONE',  ( 6.146657985744592735E-16, 3.905054717696927382E-31, 1.000000000000000000 ) ) ;
#18642=DIRECTION ( 'NONE',  ( -1.000000000000000000, 0.000000000000000000, 0.000000000000000000 ) ) ;
#18643=ORIENTED_EDGE ( 'NONE', *, *, #914, .F. ) ;
#18647=AXIS2_PLACEMENT_3D ( 'NONE', #3749, #16706, #25876 ) ;
#18651=ADVANCED_FACE ( 'NONE', ( #2132 ), #11914, .T. ) ;
#18657=DIRECTION ( 'NONE',  ( 0.000000000000000000, 0.000000000000000000, -1.000000000000000000 ) ) ;
#18659=VERTEX_POINT ( 'NONE', #8724 ) ;
#18668=CYLINDRICAL_SURFACE ( 'NONE', #25393, 1.270000000000000240 ) ;
#18670=CARTESIAN_POINT ( 'NONE',  ( 6.073982626571928556, 78.87340550758391089, 4.346604155593825958 ) ) ;
#18671=DIRECTION ( 'NONE',  ( -0.8138664877804110409, 0.5810519254489896479, 0.000000000000000000 ) ) ;
#18689=CARTESIAN_POINT ( 'NONE',  ( 5.511339492779238292, 57.14999999999997016, 5.111277471990169907 ) ) ;
#18695=ORIENTED_EDGE ( 'NONE', *, *, #28163, .F. ) ;
#18700=ORIENTED_EDGE ( 'NONE', *, *, #22369, .F. ) ;
#18707=CARTESIAN_POINT ( 'NONE',  ( 14.95453923199683111, 61.75387968257833649, -5.016499999999999737 ) ) ;
#18711=CARTESIAN_POINT ( 'NONE',  ( -5.177913976931287188, 57.15000000000002700, -5.372100000000004094 ) ) ;
#18713=CARTESIAN_POINT ( 'NONE',  ( 5.777868923222713171, 78.89722547516475970, 5.030779815616707396 ) ) ;
#18714=B_SPLINE_CURVE_WITH_KNOTS ( 'NONE', 3,
 ( #15530, #28320, #31726, #5341 ),
 .UNSPECIFIED., .F., .F.,
 ( 4, 4 ),
 ( 0.4905041263739809976, 1.000000000000000000 ),
 .UNSPECIFIED. ) ;
#18717=DIRECTION ( 'NONE',  ( 9.627370216492862708E-17, 1.000000000000000000, -0.000000000000000000 ) ) ;
#18729=CARTESIAN_POINT ( 'NONE',  ( -5.871452009091383317, 57.14999999999997016, -5.016499999999999737 ) ) ;
#18745=EDGE_CURVE ( 'NONE', #22648, #15317, #13688, .T. ) ;
#18746=VERTEX_POINT ( 'NONE', #35133 ) ;
#18747=VERTEX_POINT ( 'NONE', #5960 ) ;
#18761=CARTESIAN_POINT ( 'NONE',  ( 1.247998466936322838E-15, 12.96302561210691806, 0.000000000000000000 ) ) ;
#18764=B_SPLINE_CURVE_WITH_KNOTS ( 'NONE', 3,
 ( #22408, #33084, #3274, #83, #15821, #19228, #37870, #21657, #34682, #8904 ),
 .UNSPECIFIED., .F., .F.,
 ( 4, 2, 2, 2, 4 ),
 ( -0.0004895961982421346420, 0.0005229314014804247769, 0.001535459001202984196, 0.002547986600925542747, 0.003560514200648101299 ),
 .UNSPECIFIED. ) ;
#18768=DIRECTION ( 'NONE',  ( 0.000000000000000000, 1.000000000000000000, 0.000000000000000000 ) ) ;
#18773=ADVANCED_FACE ( 'NONE', ( #37476 ), #2350, .T. ) ;
#18782=CARTESIAN_POINT ( 'NONE',  ( 4.997525182441555636, 56.61525291752811029, -5.184946129310890051 ) ) ;
#18794=AXIS2_PLACEMENT_3D ( 'NONE', #25762, #32579, #25354 ) ;
#18800=CARTESIAN_POINT ( 'NONE',  ( -13.85159022459153988, 59.63164443796365077, -5.016499999999999737 ) ) ;
#18808=B_SPLINE_CURVE_WITH_KNOTS ( 'NONE', 3,
 ( #2274, #2696, #28021, #8224 ),
 .UNSPECIFIED., .F., .F.,
 ( 4, 4 ),
 ( 0.000000000000000000, 0.9716897010375963317 ),
 .UNSPECIFIED. ) ;
#18813=VECTOR ( 'NONE', #39209, 1000.000000000000000 ) ;
#18818=CARTESIAN_POINT ( 'NONE',  ( 20.83467972660109169, 65.95194780259438971, -5.016499999999999737 ) ) ;
#18820=VECTOR ( 'NONE', #34870, 1000.000000000000114 ) ;
#18836=ORIENTED_EDGE ( 'NONE', *, *, #2411, .T. ) ;
#18839=DIRECTION ( 'NONE',  ( 0.9849462604886047856, 0.000000000000000000, -0.1728608224830407714 ) ) ;
#18873=DIRECTION ( 'NONE',  ( 9.627370216492862708E-17, 1.000000000000000000, -0.000000000000000000 ) ) ;
#18879=CARTESIAN_POINT ( 'NONE',  ( 5.177913976931208140, 56.51499999999997925, -5.372099999999992548 ) ) ;
#18882=EDGE_CURVE ( 'NONE', #12419, #36071, #37978, .T. ) ;
#18907=COLOUR_RGB ( '', 0.08235294, 0.09019608, 0.10196078) ;
#18913=VECTOR ( 'NONE', #10392, 1000.000000000000114 ) ;
#18916=ORIENTED_EDGE ( 'NONE', *, *, #7992, .F. ) ;
#18923=DIRECTION ( 'NONE',  ( -1.000000000000000000, 0.000000000000000000, 0.000000000000000000 ) ) ;
#18924=CARTESIAN_POINT ( 'NONE',  ( -11.58677707360137354, 55.24499999999999034, 4.474811398758258285 ) ) ;
#18926=CARTESIAN_POINT ( 'NONE',  ( 5.583532163259939729, 78.91300747758680245, 5.082153855702582490 ) ) ;
#18930=CARTESIAN_POINT ( 'NONE',  ( -10.92199999999999704, 55.24499999999999034, 0.000000000000000000 ) ) ;
#18939=CIRCLE ( 'NONE', #8076, 14.73199999999999577 ) ;
#18947=LINE ( 'NONE', #6189, #40514 ) ;
#18948=FACE_OUTER_BOUND ( 'NONE', #22826, .T. ) ;
#18952=VERTEX_POINT ( 'NONE', #32989 ) ;
#18959=ORIENTED_EDGE ( 'NONE', *, *, #21198, .T. ) ;
#18968=DIRECTION ( 'NONE',  ( -0.000000000000000000, -0.000000000000000000, -1.000000000000000000 ) ) ;
#18976=CIRCLE ( 'NONE', #33259, 2.540000000000000480 ) ;
#19002=ORIENTED_EDGE ( 'NONE', *, *, #25311, .F. ) ;
#19019=VERTEX_POINT ( 'NONE', #26367 ) ;
#19024=EDGE_CURVE ( 'NONE', #24258, #31942, #29135, .T. ) ;
#19034=VERTEX_POINT ( 'NONE', #29783 ) ;
#19039=LINE ( 'NONE', #28431, #21484 ) ;
#19052=CARTESIAN_POINT ( 'NONE',  ( 4.880629475852391153, 56.51998046905271877, -4.886937129244065758 ) ) ;
#19058=DIRECTION ( 'NONE',  ( -1.000000000000000000, 0.000000000000000000, 0.000000000000000000 ) ) ;
#19059=DIRECTION ( 'NONE',  ( -0.7071067811865480168, -0.7071067811865470176, 8.659560562354937789E-17 ) ) ;
#19062=ORIENTED_EDGE ( 'NONE', *, *, #1463, .F. ) ;
#19074=ADVANCED_FACE ( 'NONE', ( #28927 ), #9347, .T. ) ;
#19084=CARTESIAN_POINT ( 'NONE',  ( -5.177913976931287188, 56.99702125087951288, 5.372100000000003206 ) ) ;
#19094=ORIENTED_EDGE ( 'NONE', *, *, #27961, .F. ) ;
#19110=EDGE_CURVE ( 'NONE', #296, #19469, #21165, .T. ) ;
#19113=LINE ( 'NONE', #35743, #4595 ) ;
#19115=VECTOR ( 'NONE', #16622, 1000.000000000000000 ) ;
#19118=EDGE_LOOP ( 'NONE', ( #39349, #3062, #22674, #4845, #9751, #19145, #33371, #30913 ) ) ;
#19123=EDGE_CURVE ( 'NONE', #19747, #5873, #4655, .T. ) ;
#19131=AXIS2_PLACEMENT_3D ( 'NONE', #31545, #8128, #21103 ) ;
#19136=CARTESIAN_POINT ( 'NONE',  ( -14.24929227862422820, 61.25037559889041461, 5.016500000000000625 ) ) ;
#19137=VECTOR ( 'NONE', #7631, 1000.000000000000114 ) ;
#19145=ORIENTED_EDGE ( 'NONE', *, *, #23354, .T. ) ;
#19146=CARTESIAN_POINT ( 'NONE',  ( -5.177913976931295181, 71.67999986514566046, 5.372100000000000541 ) ) ;
#19150=AXIS2_PLACEMENT_3D ( 'NONE', #17109, #18149, #41603 ) ;
#19155=DIRECTION ( 'NONE',  ( 0.1715592850456333363, 0.1224830539174543431, -0.9775302108976914317 ) ) ;
#19158=FILL_AREA_STYLE ('',( #2792 ) ) ;
#19171=ORIENTED_EDGE ( 'NONE', *, *, #9933, .F. ) ;
#19177=CARTESIAN_POINT ( 'NONE',  ( 10.92199999999999704, 57.14999999999999858, -4.381499999999999950 ) ) ;
#19186=ORIENTED_EDGE ( 'NONE', *, *, #12125, .T. ) ;
#19189=CARTESIAN_POINT ( 'NONE',  ( 6.905624999999943725, 85.80437499999999318, 0.000000000000000000 ) ) ;
#19194=CIRCLE ( 'NONE', #4274, 6.350000000000004974 ) ;
#19196=CARTESIAN_POINT ( 'NONE',  ( 1.172031118611134874E-15, 12.17394877578616885, 0.000000000000000000 ) ) ;
#19202=DIRECTION ( 'NONE',  ( -0.000000000000000000, -0.000000000000000000, -1.000000000000000000 ) ) ;
#19206=CYLINDRICAL_SURFACE ( 'NONE', #29349, 16.60960244842765832 ) ;
#19223=DIRECTION ( 'NONE',  ( 0.000000000000000000, 0.000000000000000000, 1.000000000000000000 ) ) ;
#19228=CARTESIAN_POINT ( 'NONE',  ( -6.604684614741059612, 78.82897922428260529, 3.487443616724451356 ) ) ;
#19233=EDGE_LOOP ( 'NONE', ( #40659, #28221, #16056, #18024, #4398, #39535, #25294, #1327 ) ) ;
#19252=DIRECTION ( 'NONE',  ( -1.000000000000000000, -6.353134868986659519E-16, 0.000000000000000000 ) ) ;
#19253=CARTESIAN_POINT ( 'NONE',  ( -5.871452009091403745, 88.73331249999999670, -5.016499999999999737 ) ) ;
#19260=EDGE_LOOP ( 'NONE', ( #4828, #4950, #32175, #8862 ) ) ;
#19266=CIRCLE ( 'NONE', #33580, 18.32410244842765934 ) ;
#19273=CYLINDRICAL_SURFACE ( 'NONE', #39065, 18.32410244842765934 ) ;
#19277=CARTESIAN_POINT ( 'NONE',  ( -10.38331224698210420, 56.51499999999998636, 4.381499999999999950 ) ) ;
#19289=CIRCLE ( 'NONE', #5721, 14.91798719394653716 ) ;
#19292=VERTEX_POINT ( 'NONE', #27006 ) ;
#19302=EDGE_CURVE ( 'NONE', #22885, #26876, #13799, .T. ) ;
#19310=CARTESIAN_POINT ( 'NONE',  ( 6.059261036834405978, 56.98375738874752727, -5.016499999999998849 ) ) ;
#19317=LINE ( 'NONE', #28286, #38469 ) ;
#19323=CARTESIAN_POINT ( 'NONE',  ( 4.781543117820231004, 56.51500000000001478, 4.872198453344559255 ) ) ;
#19330=CARTESIAN_POINT ( 'NONE',  ( -3.590790587123838709E-14, 56.51998046905274009, 0.000000000000000000 ) ) ;
#19334=CARTESIAN_POINT ( 'NONE',  ( 5.137966006445064515, 56.84472104120882108, 5.330653870689094020 ) ) ;
#19335=CARTESIAN_POINT ( 'NONE',  ( -12.21488373879589240, 71.11999999999999034, 4.381499999999999950 ) ) ;
#19340=DIRECTION ( 'NONE',  ( 1.000000000000000000, -5.463695987328526437E-16, 0.000000000000000000 ) ) ;
#19348=DIRECTION ( 'NONE',  ( 0.000000000000000000, 0.000000000000000000, 1.000000000000000000 ) ) ;
#19351=DIRECTION ( 'NONE',  ( -0.5810519254489896479, 0.8138664877804110409, 0.000000000000000000 ) ) ;
#19352=EDGE_CURVE ( 'NONE', #31634, #25703, #36602, .T. ) ;
#19361=CARTESIAN_POINT ( 'NONE',  ( 14.94465077092626970, 61.74681991364688827, 5.072843609925764774 ) ) ;
#19368=ORIENTED_EDGE ( 'NONE', *, *, #33617, .T. ) ;
#19376=VERTEX_POINT ( 'NONE', #37024 ) ;
#19386=CARTESIAN_POINT ( 'NONE',  ( -17.14499999999999957, 71.11999999999999034, -1.904999999999999583 ) ) ;
#19420=CARTESIAN_POINT ( 'NONE',  ( -5.309060684617390516E-14, 83.56599999999998829, 0.000000000000000000 ) ) ;
#19430=CARTESIAN_POINT ( 'NONE',  ( -14.60500000000000043, 71.11999999999999034, -1.904999999999999583 ) ) ;
#19432=B_SPLINE_SURFACE_WITH_KNOTS ( 'NONE', 5, 3, ( 
 ( #6697, #532, #32895, #29480 ),
 ( #13074, #13505, #38862, #112 ),
 ( #9673, #26065, #322, #26493 ),
 ( #13713, #10304, #39284, #33316 ),
 ( #39075, #9877, #39498, #39713 ),
 ( #35674, #29265, #22847, #35887 ),
 ( #3515, #13289, #26707, #26274 ),
 ( #10089, #4146, #23063, #10514 ) ),
 .UNSPECIFIED., .F., .F., .F.,
 ( 6, 2, 6 ),
 ( 4, 4 ),
 ( 0.000000000000000000, 0.5000000000000000000, 1.000000000000000000 ),
 ( -0.002373312499999994350, 0.03277393749999998884 ),
 .UNSPECIFIED. ) ;
#19446=CARTESIAN_POINT ( 'NONE',  ( 18.35410564743290962, 77.35382415001784295, -5.392902600000141433 ) ) ;
#19449=CARTESIAN_POINT ( 'NONE',  ( -19.68500000000000227, 71.11999999999999034, 5.016499999999999737 ) ) ;
#19452=LINE ( 'NONE', #9665, #41935 ) ;
#19455=CARTESIAN_POINT ( 'NONE',  ( -18.35410564743290607, 77.35382415001784295, 5.016499999999999737 ) ) ;
#19457=CARTESIAN_POINT ( 'NONE',  ( -3.745035802202505265E-14, 57.78499999999999659, -1.904999999999999805 ) ) ;
#19461=VECTOR ( 'NONE', #21928, 1000.000000000000000 ) ;
#19469=VERTEX_POINT ( 'NONE', #15471 ) ;
#19474=CARTESIAN_POINT ( 'NONE',  ( 10.92199999999999704, 55.98894877578618434, 4.336808689942017736E-15 ) ) ;
#19483=ORIENTED_EDGE ( 'NONE', *, *, #22386, .T. ) ;
#19502=CARTESIAN_POINT ( 'NONE',  ( -11.58677707360137532, 17.14500000000000313, 4.474811398758258285 ) ) ;
#19515=VECTOR ( 'NONE', #9717, 1000.000000000000000 ) ;
#19524=CARTESIAN_POINT ( 'NONE',  ( -4.792324638262704717, 56.51998046905272588, -4.972049999962482758 ) ) ;
#19541=CARTESIAN_POINT ( 'NONE',  ( -17.14499999999998892, 57.14999999999997726, -4.381499999999999950 ) ) ;
#19544=CARTESIAN_POINT ( 'NONE',  ( -5.706393392168954470, 56.51500000000000057, -5.041882957346543570 ) ) ;
#19553=ORIENTED_EDGE ( 'NONE', *, *, #2912, .T. ) ;
#19554=ORIENTED_EDGE ( 'NONE', *, *, #8720, .F. ) ;
#19568=ADVANCED_FACE ( 'NONE', ( #2078 ), #18446, .T. ) ;
#19569=CARTESIAN_POINT ( 'NONE',  ( -13.85159022459153633, 16.59642619247576789, -5.016499999999999737 ) ) ;
#19571=CARTESIAN_POINT ( 'NONE',  ( 5.460438898883120729, 56.51499999999997215, -4.448267477574868956 ) ) ;
#19575=ORIENTED_EDGE ( 'NONE', *, *, #21909, .T. ) ;
#19593=ADVANCED_FACE ( 'NONE', ( #34245 ), #28475, .T. ) ;
#19601=FACE_OUTER_BOUND ( 'NONE', #38840, .T. ) ;
#19612=CIRCLE ( 'NONE', #34602, 6.985000000000000320 ) ;
#19617=CYLINDRICAL_SURFACE ( 'NONE', #18490, 13.46199999999999442 ) ;
#19622=DIRECTION ( 'NONE',  ( -1.000000000000000000, 0.000000000000000000, -9.769962616701377556E-15 ) ) ;
#19645=ORIENTED_EDGE ( 'NONE', *, *, #25329, .F. ) ;
#19654=EDGE_CURVE ( 'NONE', #31005, #14016, #2138, .T. ) ;
#19660=VECTOR ( 'NONE', #25551, 1000.000000000000000 ) ;
#19662=CARTESIAN_POINT ( 'NONE',  ( -17.14499999999999957, 71.11999999999999034, 5.016499999999999737 ) ) ;
#19680=CARTESIAN_POINT ( 'NONE',  ( 5.153324091224940950, 56.51694919289779051, -4.640537933338372945 ) ) ;
#19687=DIRECTION ( 'NONE',  ( 9.627370216492862708E-17, 1.000000000000000000, -0.000000000000000000 ) ) ;
#19707=EDGE_CURVE ( 'NONE', #37417, #10059, #29314, .T. ) ;
#19726=ORIENTED_EDGE ( 'NONE', *, *, #1086, .T. ) ;
#19730=CARTESIAN_POINT ( 'NONE',  ( 1.332716859069107315E-15, 13.84300000000000352, 0.000000000000000000 ) ) ;
#19741=B_SPLINE_CURVE_WITH_KNOTS ( 'NONE', 3,
 ( #20442, #11288, #1519, #20653 ),
 .UNSPECIFIED., .F., .F.,
 ( 4, 4 ),
 ( 0.000000000000000000, 0.5643836377221602696 ),
 .UNSPECIFIED. ) ;
#19746=EDGE_CURVE ( 'NONE', #28439, #4652, #35293, .T. ) ;
#19747=VERTEX_POINT ( 'NONE', #19502 ) ;
#19749=CARTESIAN_POINT ( 'NONE',  ( 4.897655256226133069, 56.53910281269273241, 5.081330806033577119 ) ) ;
#19754=CARTESIAN_POINT ( 'NONE',  ( -5.941785709847915875, 56.51500000000976343, -5.016499812912763367 ) ) ;
#19755=CARTESIAN_POINT ( 'NONE',  ( -18.35410564743290607, 77.35382415001784295, -5.016499999999999737 ) ) ;
#19757=VECTOR ( 'NONE', #3321, 1000.000000000000114 ) ;
#19777=( LENGTH_UNIT ( ) NAMED_UNIT ( * ) SI_UNIT ( .MILLI., .METRE. ) );
#19801=EDGE_CURVE ( 'NONE', #40534, #5419, #39328, .T. ) ;
#19805=ORIENTED_EDGE ( 'NONE', *, *, #40737, .F. ) ;
#19809=CARTESIAN_POINT ( 'NONE',  ( 11.04921058900168873, 56.51500000000000057, -4.436160551868584712 ) ) ;
#19824=TOROIDAL_SURFACE ( 'NONE', #41633, 17.68910244842765778, 0.6350000000000000089 ) ;
#19830=DIRECTION ( 'NONE',  ( -1.000000000000000000, 9.563967653961371147E-17, 0.000000000000000000 ) ) ;
#19844=EDGE_CURVE ( 'NONE', #11444, #11585, #9605, .T. ) ;
#19856=ORIENTED_EDGE ( 'NONE', *, *, #4596, .T. ) ;
#19864=DIRECTION ( 'NONE',  ( -9.627370216492862708E-17, -1.000000000000000000, 0.000000000000000000 ) ) ;
#19865=EDGE_CURVE ( 'NONE', #12920, #38620, #32300, .T. ) ;
#19875=CARTESIAN_POINT ( 'NONE',  ( -14.60500000000000043, 71.11999999999999034, -5.016499999999999737 ) ) ;
#19876=CARTESIAN_POINT ( 'NONE',  ( 13.85159022459153988, 16.51000000000000156, 5.016499999999999737 ) ) ;
#19880=DIRECTION ( 'NONE',  ( 0.1469470846586743706, 9.335746474409589170E-17, -0.9891443546370348727 ) ) ;
#19902=CARTESIAN_POINT ( 'NONE',  ( 5.305748947172212127, 57.14999999999999858, -5.247078976224250013 ) ) ;
#19903=DIRECTION ( 'NONE',  ( 0.000000000000000000, 0.000000000000000000, 1.000000000000000000 ) ) ;
#19904=ORIENTED_EDGE ( 'NONE', *, *, #39123, .T. ) ;
#19918=ORIENTED_EDGE ( 'NONE', *, *, #86, .T. ) ;
#19939=VERTEX_POINT ( 'NONE', #39119 ) ;
#19951=CARTESIAN_POINT ( 'NONE',  ( 14.80692295515832058, 78.04183178746350791, 5.016499999999999737 ) ) ;
#19952=DIRECTION ( 'NONE',  ( -1.000000000000000000, 9.627370216492861475E-17, 0.000000000000000000 ) ) ;
#19962=CYLINDRICAL_SURFACE ( 'NONE', #14358, 0.6349999999999966782 ) ;
#19969=ORIENTED_EDGE ( 'NONE', *, *, #433, .T. ) ;
#19977=CARTESIAN_POINT ( 'NONE',  ( -5.706393392231406736, 57.14999999999999147, -5.041882957777242602 ) ) ;
#19985=CARTESIAN_POINT ( 'NONE',  ( -5.299459906814613319, 78.93540349268876355, -5.255323016343699472 ) ) ;
#19986=ORIENTED_EDGE ( 'NONE', *, *, #2083, .F. ) ;
#20029=CARTESIAN_POINT ( 'NONE',  ( 11.66725022230186859, 55.42194143536244155, 5.016499999999783910 ) ) ;
#20037=CARTESIAN_POINT ( 'NONE',  ( -10.96186877710187879, 56.39406130473896894, -5.016500000000648996 ) ) ;
#20040=CARTESIAN_POINT ( 'NONE',  ( 14.60500000000000043, 71.11999999999999034, -5.016499999999999737 ) ) ;
#20064=VERTEX_POINT ( 'NONE', #32512 ) ;
#20067=EDGE_LOOP ( 'NONE', ( #299, #26744, #37728, #9915 ) ) ;
#20085=CARTESIAN_POINT ( 'NONE',  ( -5.860205464924994168, 57.14999999999999147, 5.019550311879309668 ) ) ;
#20088=EDGE_CURVE ( 'NONE', #38242, #11659, #4685, .T. ) ;
#20109=CIRCLE ( 'NONE', #28264, 2.540000000000000480 ) ;
#20142=UNCERTAINTY_MEASURE_WITH_UNIT (LENGTH_MEASURE( 1.000000000000000082E-05 ), #38995, 'distance_accuracy_value', 'NONE');
#20144=EDGE_LOOP ( 'NONE', ( #39999, #18916, #4744, #35589 ) ) ;
#20152=EDGE_LOOP ( 'NONE', ( #18536, #11193, #3052, #11961 ) ) ;
#20166=ADVANCED_FACE ( 'NONE', ( #10186 ), #13178, .T. ) ;
#20170=DIRECTION ( 'NONE',  ( -1.000000000000000000, -9.933992704233682996E-16, 0.000000000000000000 ) ) ;
#20190=ORIENTED_EDGE ( 'NONE', *, *, #11811, .T. ) ;
#20228=EDGE_CURVE ( 'NONE', #27998, #14963, #13600, .T. ) ;
#20235=DIRECTION ( 'NONE',  ( 0.000000000000000000, 1.000000000000000000, 0.000000000000000000 ) ) ;
#20238=ORIENTED_EDGE ( 'NONE', *, *, #2488, .T. ) ;
#20242=CARTESIAN_POINT ( 'NONE',  ( -5.540303739757925783, 78.91648400349117765, 5.100389098699535495 ) ) ;
#20243=CARTESIAN_POINT ( 'NONE',  ( -10.54112285291057560, 57.14999999999385949, -5.016499999999999737 ) ) ;
#20247=CARTESIAN_POINT ( 'NONE',  ( -5.348924234571052594, 56.51499999999999346, -4.492130288940743732 ) ) ;
#20254=FACE_OUTER_BOUND ( 'NONE', #30490, .T. ) ;
#20289=CARTESIAN_POINT ( 'NONE',  ( -5.449044798801134348, 56.51500000000043400, 5.145813327035688722 ) ) ;
#20294=VERTEX_POINT ( 'NONE', #37798 ) ;
#20298=VERTEX_POINT ( 'NONE', #36407 ) ;
#20306=CARTESIAN_POINT ( 'NONE',  ( -5.451267667241070720E-14, 85.80437499999999318, 0.000000000000000000 ) ) ;
#20324=ORIENTED_EDGE ( 'NONE', *, *, #38073, .T. ) ;
#20327=CARTESIAN_POINT ( 'NONE',  ( -12.21488373879588885, 56.36092316367923871, 5.016500000000000625 ) ) ;
#20347=ORIENTED_EDGE ( 'NONE', *, *, #8174, .F. ) ;
#20358=CARTESIAN_POINT ( 'NONE',  ( 13.85159022459154876, 16.68226173831723003, 5.016499999999999737 ) ) ;
#20385=AXIS2_PLACEMENT_3D ( 'NONE', #2559, #34708, #1923 ) ;
#20396=VERTEX_POINT ( 'NONE', #22426 ) ;
#20413=CARTESIAN_POINT ( 'NONE',  ( 6.059261036834406866, 65.30181249999998272, -5.016499999999999737 ) ) ;
#20435=DIRECTION ( 'NONE',  ( 9.627370216492862708E-17, 1.000000000000000000, -0.000000000000000000 ) ) ;
#20437=( BOUNDED_CURVE ( )  B_SPLINE_CURVE ( 3, ( #39777, #13194, #41968, #12973 ),
 .UNSPECIFIED., .F., .T. ) 
 B_SPLINE_CURVE_WITH_KNOTS ( ( 4, 4 ),
 ( 4.712388980384688786, 5.673871460451329618 ),
 .UNSPECIFIED. ) 
 CURVE ( )  GEOMETRIC_REPRESENTATION_ITEM ( )  RATIONAL_B_SPLINE_CURVE ( ( 1.000000000000000000, 0.9244349266169029633, 0.9244349266169029633, 1.000000000000000000 ) ) 
 REPRESENTATION_ITEM ( '' )  );
#20442=CARTESIAN_POINT ( 'NONE',  ( 18.35410564743290607, 77.35382415001784295, -5.016499999999999737 ) ) ;
#20467=AXIS2_PLACEMENT_3D ( 'NONE', #10273, #3698, #17081 ) ;
#20484=CARTESIAN_POINT ( 'NONE',  ( 11.32678463655022405, 56.02547433970799773, -4.456118031212427333 ) ) ;
#20489=VECTOR ( 'NONE', #19880, 1000.000000000000114 ) ;
#20497=ORIENTED_EDGE ( 'NONE', *, *, #41421, .T. ) ;
#20510=EDGE_LOOP ( 'NONE', ( #16556, #15086, #11564, #20497, #8024 ) ) ;
#20541=CARTESIAN_POINT ( 'NONE',  ( -5.137966006445163991, 56.84472104120892055, -5.330653870689114449 ) ) ;
#20549=CARTESIAN_POINT ( 'NONE',  ( 6.059261036834406866, 57.14999999999999858, 5.016499999999999737 ) ) ;
#20563=PLANE ( 'NONE',  #12491 ) ;
#20572=CARTESIAN_POINT ( 'NONE',  ( -18.13811525448111439, 9.293884745518889545, 2.221278478896607584E-15 ) ) ;
#20581=VERTEX_POINT ( 'NONE', #19876 ) ;
#20586=ORIENTED_EDGE ( 'NONE', *, *, #19801, .T. ) ;
#20612=DIRECTION ( 'NONE',  ( -1.000000000000000000, 0.000000000000000000, -1.776356839400250465E-15 ) ) ;
#20643=ORIENTED_EDGE ( 'NONE', *, *, #38355, .F. ) ;
#20647=AXIS2_PLACEMENT_3D ( 'NONE', #22864, #2895, #38875 ) ;
#20649=CARTESIAN_POINT ( 'NONE',  ( 12.21488373879589062, 56.36092316367926003, 5.016499999999999737 ) ) ;
#20653=CARTESIAN_POINT ( 'NONE',  ( 6.059261036833980540, 78.87450423423040036, -5.016499999999999737 ) ) ;
#20657=DIRECTION ( 'NONE',  ( 1.000000000000000000, -1.177520686924251719E-16, 0.000000000000000000 ) ) ;
#20666=CARTESIAN_POINT ( 'NONE',  ( -5.714078020758869059, 78.90256189635195483, 5.042866571093570727 ) ) ;
#20671=CARTESIAN_POINT ( 'NONE',  ( -4.792324638262704717, 56.51998046905272588, -4.972049999962482758 ) ) ;
#20684=ORIENTED_EDGE ( 'NONE', *, *, #2411, .F. ) ;
#20706=EDGE_CURVE ( 'NONE', #24253, #1422, #20971, .T. ) ;
#20713=DIRECTION ( 'NONE',  ( -0.1715592850456333363, -0.1224830539174543431, -0.9775302108976914317 ) ) ;
#20727=CARTESIAN_POINT ( 'NONE',  ( 6.349999999999945466, 86.35999999999998522, 0.000000000000000000 ) ) ;
#20768=ORIENTED_EDGE ( 'NONE', *, *, #28163, .T. ) ;
#20784=ORIENTED_EDGE ( 'NONE', *, *, #15180, .F. ) ;
#20797=DIRECTION ( 'NONE',  ( 9.627370216492862708E-17, 1.000000000000000000, -0.000000000000000000 ) ) ;
#20799=ORIENTED_EDGE ( 'NONE', *, *, #26054, .T. ) ;
#20806=FACE_OUTER_BOUND ( 'NONE', #10482, .T. ) ;
#20808=CYLINDRICAL_SURFACE ( 'NONE', #899, 0.6350000000000001199 ) ;
#20816=ORIENTED_EDGE ( 'NONE', *, *, #27463, .F. ) ;
#20824=CONICAL_SURFACE ( 'NONE', #21482, 12.69999999999999751, 0.7853981633974471688 ) ;
#20825=ORIENTED_EDGE ( 'NONE', *, *, #23992, .F. ) ;
#20835=CARTESIAN_POINT ( 'NONE',  ( 5.177913976931209916, 65.30181249999998272, -5.372099999999993436 ) ) ;
#20862=DIRECTION ( 'NONE',  ( 9.627370216492862708E-17, 1.000000000000000000, -0.000000000000000000 ) ) ;
#20868=EDGE_LOOP ( 'NONE', ( #41826, #2216, #41441, #27180 ) ) ;
#20892=EDGE_LOOP ( 'NONE', ( #19483, #841, #24568, #26076, #40984 ) ) ;
#20897=CARTESIAN_POINT ( 'NONE',  ( -5.348924234571056147, 56.51499999999999346, 4.492130288940740179 ) ) ;
#20903=EDGE_CURVE ( 'NONE', #11738, #32240, #6053, .T. ) ;
#20918=CARTESIAN_POINT ( 'NONE',  ( -11.42297701379735564, 55.88459609804033335, 4.463034230327252772 ) ) ;
#20945=CARTESIAN_POINT ( 'NONE',  ( 6.059261036834406866, 56.51500000000000057, 4.547742611252461487 ) ) ;
#20953=EDGE_CURVE ( 'NONE', #20294, #1007, #23912, .T. ) ;
#20956=ORIENTED_EDGE ( 'NONE', *, *, #8411, .T. ) ;
#20971=CIRCLE ( 'NONE', #26429, 6.350000000000004974 ) ;
#20972=CARTESIAN_POINT ( 'NONE',  ( 5.241362157049057835, 57.14999999999998437, 5.310945289804168468 ) ) ;
#20974=DIRECTION ( 'NONE',  ( -6.353134868986659519E-16, 1.000000000000000000, 0.000000000000000000 ) ) ;
#20977=VERTEX_POINT ( 'NONE', #40548 ) ;
#20994=LINE ( 'NONE', #40206, #27195 ) ;
#20995=EDGE_LOOP ( 'NONE', ( #25128, #14404 ) ) ;
#21005=VERTEX_POINT ( 'NONE', #24122 ) ;
#21009=CARTESIAN_POINT ( 'NONE',  ( 13.85159022459153988, 16.51000000000000156, -5.016499999999999737 ) ) ;
#21018=CARTESIAN_POINT ( 'NONE',  ( 6.059261036834405978, 56.51500000000000057, 4.381499999999999950 ) ) ;
#21025=DIRECTION ( 'NONE',  ( -6.353134868986659519E-16, 1.000000000000000000, 0.000000000000000000 ) ) ;
#21037=ORIENTED_EDGE ( 'NONE', *, *, #22706, .F. ) ;
#21058=VERTEX_POINT ( 'NONE', #8155 ) ;
#21064=VERTEX_POINT ( 'NONE', #37132 ) ;
#21067=CIRCLE ( 'NONE', #15623, 0.6350000000000001199 ) ;
#21071=DIRECTION ( 'NONE',  ( -1.000000000000000000, 0.000000000000000000, 0.000000000000000000 ) ) ;
#21073=LINE ( 'NONE', #8100, #14032 ) ;
#21082=DIRECTION ( 'NONE',  ( -0.000000000000000000, -0.000000000000000000, -1.000000000000000000 ) ) ;
#21103=DIRECTION ( 'NONE',  ( -1.000000000000000000, 1.044409991968846932E-16, 0.000000000000000000 ) ) ;
#21107=CARTESIAN_POINT ( 'NONE',  ( 11.04921058900168518, 56.51500000000000057, 4.436160551868583823 ) ) ;
#21113=CARTESIAN_POINT ( 'NONE',  ( 10.54112285291057916, 57.14999999999387370, -5.016500000000000625 ) ) ;
#21121=CARTESIAN_POINT ( 'NONE',  ( -11.66725022230187214, 55.42194143536246287, 5.016499999999784798 ) ) ;
#21122=EDGE_CURVE ( 'NONE', #18118, #20396, #27853, .T. ) ;
#21135=DIRECTION ( 'NONE',  ( 0.1469470846586743706, 9.335746474409589170E-17, -0.9891443546370348727 ) ) ;
#21146=EDGE_LOOP ( 'NONE', ( #4003, #33710, #34346, #4019 ) ) ;
#21147=CARTESIAN_POINT ( 'NONE',  ( 6.059261036834405978, 56.51500000000000057, 4.381499999999999950 ) ) ;
#21156=VERTEX_POINT ( 'NONE', #38082 ) ;
#21165=CIRCLE ( 'NONE', #6245, 16.60960244842765832 ) ;
#21170=EDGE_CURVE ( 'NONE', #38620, #33803, #29875, .T. ) ;
#21179=ORIENTED_EDGE ( 'NONE', *, *, #12597, .F. ) ;
#21192=CARTESIAN_POINT ( 'NONE',  ( 6.984999999999963904, 56.51500000000000057, 8.554157892044261576E-16 ) ) ;
#21197=DIRECTION ( 'NONE',  ( 0.000000000000000000, 0.000000000000000000, -1.000000000000000000 ) ) ;
#21198=EDGE_CURVE ( 'NONE', #26767, #12920, #9459, .T. ) ;
#21211=CARTESIAN_POINT ( 'NONE',  ( 13.85159022459154876, 16.68226173831723003, -5.016499999999999737 ) ) ;
#21214=ORIENTED_EDGE ( 'NONE', *, *, #39678, .T. ) ;
#21238=DIRECTION ( 'NONE',  ( -9.627370216492862708E-17, -1.000000000000000000, 0.000000000000000000 ) ) ;
#21240=ORIENTED_EDGE ( 'NONE', *, *, #12698, .F. ) ;
#21257=ORIENTED_EDGE ( 'NONE', *, *, #27362, .F. ) ;
#21264=AXIS2_PLACEMENT_3D ( 'NONE', #6748, #35298, #32952 ) ;
#21273=DIRECTION ( 'NONE',  ( 0.000000000000000000, -1.000000000000000000, 0.000000000000000000 ) ) ;
#21279=DIRECTION ( 'NONE',  ( -0.000000000000000000, -0.000000000000000000, -1.000000000000000000 ) ) ;
#21280=DIRECTION ( 'NONE',  ( 5.463695987328526437E-16, -1.000000000000000000, -1.672774450599033775E-31 ) ) ;
#21283=ORIENTED_EDGE ( 'NONE', *, *, #11250, .T. ) ;
#21288=DIRECTION ( 'NONE',  ( -6.146657985744592735E-16, 3.905054717696928257E-31, 1.000000000000000000 ) ) ;
#21316=AXIS2_PLACEMENT_3D ( 'NONE', #7416, #33399, #20170 ) ;
#21320=CARTESIAN_POINT ( 'NONE',  ( 11.55299880265467571, 55.57741982016698046, -4.472382752598256239 ) ) ;
#21341=ORIENTED_EDGE ( 'NONE', *, *, #22509, .F. ) ;
#21343=ORIENTED_EDGE ( 'NONE', *, *, #2757, .F. ) ;
#21354=PLANE ( 'NONE',  #38637 ) ;
#21373=DIRECTION ( 'NONE',  ( -1.000000000000000000, 0.000000000000000000, 0.000000000000000000 ) ) ;
#21382=VERTEX_POINT ( 'NONE', #32523 ) ;
#21386=ORIENTED_EDGE ( 'NONE', *, *, #15412, .F. ) ;
#21408=ADVANCED_BREP_SHAPE_REPRESENTATION ( '', ( #38952, #3275 ), #40037 ) ;
#21416=DIRECTION ( 'NONE',  ( 0.1715592850456333085, -0.1224830539174543292, -0.9775302108976914317 ) ) ;
#21441=CARTESIAN_POINT ( 'NONE',  ( 1.589478822742971486E-15, 16.51000000000000156, 0.000000000000000000 ) ) ;
#21446=CARTESIAN_POINT ( 'NONE',  ( 5.177913976931196594, 78.94499979771845233, -5.372100000000001430 ) ) ;
#21465=ORIENTED_EDGE ( 'NONE', *, *, #877, .T. ) ;
#21482=AXIS2_PLACEMENT_3D ( 'NONE', #25510, #15699, #15497 ) ;
#21484=VECTOR ( 'NONE', #42072, 1000.000000000000000 ) ;
#21492=LINE ( 'NONE', #17680, #18090 ) ;
#21547=CARTESIAN_POINT ( 'NONE',  ( 15.15189561879764746, 77.97492127061565270, -1.904999999999999583 ) ) ;
#21554=CARTESIAN_POINT ( 'NONE',  ( -14.73199999999999932, 12.96416000000000146, 0.000000000000000000 ) ) ;
#21573=ORIENTED_EDGE ( 'NONE', *, *, #4113, .F. ) ;
#21589=CARTESIAN_POINT ( 'NONE',  ( -5.241362157049148429, 77.01756249999996840, -5.310945289804168468 ) ) ;
#21610=CARTESIAN_POINT ( 'NONE',  ( -5.460472493305379871, 56.51500000000001478, -4.448254263655326390 ) ) ;
#21638=EDGE_CURVE ( 'NONE', #32351, #18952, #38027, .T. ) ;
#21639=CARTESIAN_POINT ( 'NONE',  ( 6.059261036834405978, 56.51500000000000057, -4.381499999999999950 ) ) ;
#21643=ADVANCED_FACE ( 'NONE', ( #34837 ), #40808, .T. ) ;
#21644=DIRECTION ( 'NONE',  ( 1.000000000000000000, -1.162840169671635117E-16, 0.000000000000000000 ) ) ;
#21647=ORIENTED_EDGE ( 'NONE', *, *, #18057, .F. ) ;
#21657=CARTESIAN_POINT ( 'NONE',  ( -7.019433301159665461, 78.79326733250417192, 2.552382320839211349 ) ) ;
#21659=DIRECTION ( 'NONE',  ( 1.000000000000000000, 0.000000000000000000, -5.975917486140574681E-16 ) ) ;
#21687=ADVANCED_FACE ( 'NONE', ( #2260 ), #12033, .T. ) ;
#21689=VECTOR ( 'NONE', #28116, 1000.000000000000000 ) ;
#21690=CARTESIAN_POINT ( 'NONE',  ( 6.059261036833980540, 78.87450423423040036, -5.016499999999999737 ) ) ;
#21695=ORIENTED_EDGE ( 'NONE', *, *, #5067, .T. ) ;
#21702=DIRECTION ( 'NONE',  ( -1.000000000000000000, 0.000000000000000000, 0.000000000000000000 ) ) ;
#21707=DIRECTION ( 'NONE',  ( 1.000000000000000000, -9.627370216492862708E-17, 0.000000000000000000 ) ) ;
#21734=CARTESIAN_POINT ( 'NONE',  ( -18.32410244842765934, 8.844871939465427602, 0.000000000000000000 ) ) ;
#21757=DIRECTION ( 'NONE',  ( 0.000000000000000000, 0.000000000000000000, 1.000000000000000000 ) ) ;
#21759=CARTESIAN_POINT ( 'NONE',  ( -17.14499999999999957, 71.11999999999999034, 5.016499999999999737 ) ) ;
#21762=ORIENTED_EDGE ( 'NONE', *, *, #16452, .T. ) ;
#21769=AXIS2_PLACEMENT_3D ( 'NONE', #22817, #33076, #36687 ) ;
#21778=CARTESIAN_POINT ( 'NONE',  ( -16.60960244842765832, 9.026346327358517385, 2.034089647357696937E-15 ) ) ;
#21793=( BOUNDED_SURFACE ( )  B_SPLINE_SURFACE ( 3, 2, ( 
 ( #3719, #29682, #14314 ),
 ( #28530, #41746, #31936 ),
 ( #30722, #14529, #11342 ),
 ( #15526, #15312, #24328 ),
 ( #41535, #37128, #31722 ),
 ( #37334, #31507, #41326 ),
 ( #38121, #40545, #20918 ),
 ( #2354, #33941, #11132 ),
 ( #22314, #21121, #2771 ),
 ( #27538, #28733, #18924 ) ),
 .UNSPECIFIED., .F., .F., .T. ) 
 B_SPLINE_SURFACE_WITH_KNOTS ( ( 4, 2, 2, 2, 4 ),
 ( 3, 3 ),
 ( 1.570796326794897002, 1.963495408493620920, 2.356194490192344837, 2.748893571891068532, 3.141592653589792672 ),
 ( 0.000000000000000000, 1.000000000000000000 ),
 .UNSPECIFIED. ) 
 GEOMETRIC_REPRESENTATION_ITEM ( )  RATIONAL_B_SPLINE_SURFACE ( (
 ( 1.000000000000000000, 0.7071067811865475727, 1.000000000000000000),
 ( 1.000000000000000000, 0.7139102541735814489, 1.000000000000000000),
 ( 1.000000000000000000, 0.7206031636706378141, 1.000000000000000000),
 ( 1.000000000000000000, 0.7328301610699465840, 1.000000000000000000),
 ( 1.000000000000000000, 0.7383589052090805405, 1.000000000000000000),
 ( 1.000000000000000000, 0.7475127447242121415, 1.000000000000000000),
 ( 1.000000000000000000, 0.7511365686956648080, 1.000000000000000000),
 ( 1.000000000000000000, 0.7560206254140624527, 1.000000000000000000),
 ( 1.000000000000000000, 0.7572851909592275277, 1.000000000000000000),
 ( 1.000000000000000000, 0.7572803591334833495, 1.000000000000000000) ) ) 
 REPRESENTATION_ITEM ( '' )  SURFACE ( )  );
#21804=CARTESIAN_POINT ( 'NONE',  ( -5.177913976931302287, 77.01756249999996840, -5.372099999999996989 ) ) ;
#21817=CARTESIAN_POINT ( 'NONE',  ( 5.477532837487817829, 78.92140300690502386, -5.132221182818687666 ) ) ;
#21838=CARTESIAN_POINT ( 'NONE',  ( -10.28897677580358305, 56.51499999999998636, -4.381499999999999950 ) ) ;
#21840=ORIENTED_EDGE ( 'NONE', *, *, #2521, .T. ) ;
#21844=CARTESIAN_POINT ( 'NONE',  ( 17.14499999999999957, 71.11999999999999034, 5.016499999999999737 ) ) ;
#21848=DIRECTION ( 'NONE',  ( -0.8138664877804110409, -0.5810519254489896479, 0.000000000000000000 ) ) ;
#21872=CARTESIAN_POINT ( 'NONE',  ( 6.072850655491107474, 78.87349744216250258, -4.348040511725084656 ) ) ;
#21892=ORIENTED_EDGE ( 'NONE', *, *, #392, .F. ) ;
#21908=DIRECTION ( 'NONE',  ( -1.000000000000000000, 0.000000000000000000, -6.146657985744586818E-16 ) ) ;
#21909=EDGE_CURVE ( 'NONE', #10948, #5725, #39882, .T. ) ;
#21912=ORIENTED_EDGE ( 'NONE', *, *, #18882, .T. ) ;
#21928=DIRECTION ( 'NONE',  ( 0.000000000000000000, 1.000000000000000000, 0.000000000000000000 ) ) ;
#21938=AXIS2_PLACEMENT_3D ( 'NONE', #37226, #30617, #1460 ) ;
#21943=FACE_OUTER_BOUND ( 'NONE', #16287, .T. ) ;
#21947=CARTESIAN_POINT ( 'NONE',  ( -17.14499999999999957, 71.11999999999999034, 5.016499999999999737 ) ) ;
#21950=ADVANCED_FACE ( 'NONE', ( #26451 ), #10678, .F. ) ;
#21956=DIRECTION ( 'NONE',  ( -0.9891443546370349837, 0.000000000000000000, 0.1469470846586743984 ) ) ;
#21957=VECTOR ( 'NONE', #35417, 1000.000000000000227 ) ;
#21967=ADVANCED_FACE ( 'NONE', ( #18948 ), #41348, .F. ) ;
#21980=VERTEX_POINT ( 'NONE', #35360 ) ;
#22014=VECTOR ( 'NONE', #22427, 1000.000000000000000 ) ;
#22021=DIRECTION ( 'NONE',  ( 9.627370216492862708E-17, 1.000000000000000000, -0.000000000000000000 ) ) ;
#22024=ORIENTED_EDGE ( 'NONE', *, *, #21170, .T. ) ;
#22047=VECTOR ( 'NONE', #970, 1000.000000000000114 ) ;
#22068=CARTESIAN_POINT ( 'NONE',  ( 4.781529118576645310, 56.51499999999997215, -4.872211946655240489 ) ) ;
#22071=CARTESIAN_POINT ( 'NONE',  ( -5.511275327887647180, 56.51499999999913371, 5.111309966001401861 ) ) ;
#22073=ORIENTED_EDGE ( 'NONE', *, *, #21638, .F. ) ;
#22084=FACE_OUTER_BOUND ( 'NONE', #37144, .T. ) ;
#22105=LINE ( 'NONE', #12542, #5521 ) ;
#22124=CARTESIAN_POINT ( 'NONE',  ( 5.266289895157169814E-14, 83.56599999999998829, 1.904999999999999805 ) ) ;
#22158=EDGE_CURVE ( 'NONE', #38242, #22885, #33987, .T. ) ;
#22173=DIRECTION ( 'NONE',  ( 1.000000000000000000, 5.463695987328526437E-16, -6.146657985744592735E-16 ) ) ;
#22181=ORIENTED_EDGE ( 'NONE', *, *, #18043, .T. ) ;
#22184=ORIENTED_EDGE ( 'NONE', *, *, #31090, .T. ) ;
#22185=LINE ( 'NONE', #21554, #21957 ) ;
#22192=ORIENTED_EDGE ( 'NONE', *, *, #33225, .T. ) ;
#22208=FACE_OUTER_BOUND ( 'NONE', #20892, .T. ) ;
#22211=LINE ( 'NONE', #19449, #30763 ) ;
#22224=CARTESIAN_POINT ( 'NONE',  ( -5.305748947172281405, 53.58606249999999704, -5.247078976224250013 ) ) ;
#22242=CARTESIAN_POINT ( 'NONE',  ( 17.14499999999999957, 71.11999999999999034, 5.016499999999999737 ) ) ;
#22246=CARTESIAN_POINT ( 'NONE',  ( -3.630816577625875226E-14, 57.14999999999999147, 0.000000000000000000 ) ) ;
#22249=ORIENTED_EDGE ( 'NONE', *, *, #3477, .F. ) ;
#22258=CIRCLE ( 'NONE', #31022, 2.540000000000000480 ) ;
#22281=CARTESIAN_POINT ( 'NONE',  ( 6.059261036833978764, 78.87450423423040036, 5.016499999999999737 ) ) ;
#22295=CARTESIAN_POINT ( 'NONE',  ( 5.177913976931197482, 56.51500000000002188, 5.372099999999984554 ) ) ;
#22301=ORIENTED_EDGE ( 'NONE', *, *, #19123, .F. ) ;
#22309=CYLINDRICAL_SURFACE ( 'NONE', #9971, 0.6349999999999966782 ) ;
#22314=CARTESIAN_POINT ( 'NONE',  ( -12.21488373878702127, 55.49440886859295574, 5.016499999999999737 ) ) ;
#22323=CARTESIAN_POINT ( 'NONE',  ( -5.177913976931285411, 57.14999999999998437, 5.372100000000002318 ) ) ;
#22328=AXIS2_PLACEMENT_3D ( 'NONE', #22242, #25872, #35905 ) ;
#22347=ORIENTED_EDGE ( 'NONE', *, *, #20088, .T. ) ;
#22361=DIRECTION ( 'NONE',  ( -0.000000000000000000, -0.000000000000000000, -1.000000000000000000 ) ) ;
#22369=EDGE_CURVE ( 'NONE', #21980, #35923, #38745, .T. ) ;
#22379=CARTESIAN_POINT ( 'NONE',  ( -10.92199999999999704, 55.24499999999999034, 0.000000000000000000 ) ) ;
#22383=CARTESIAN_POINT ( 'NONE',  ( -11.58677707360137532, 55.98894877578615592, -4.474811398758257397 ) ) ;
#22386=EDGE_CURVE ( 'NONE', #29922, #39604, #5644, .T. ) ;
#22400=ORIENTED_EDGE ( 'NONE', *, *, #24581, .F. ) ;
#22403=CARTESIAN_POINT ( 'NONE',  ( 8.689997779576109740E-16, 9.026346327358515609, 0.000000000000000000 ) ) ;
#22408=CARTESIAN_POINT ( 'NONE',  ( -5.177913976931298734, 78.94499979771843812, 5.372100000000002318 ) ) ;
#22411=ORIENTED_EDGE ( 'NONE', *, *, #21198, .F. ) ;
#22417=VECTOR ( 'NONE', #18553, 1000.000000000000114 ) ;
#22426=CARTESIAN_POINT ( 'NONE',  ( -11.66725022231030984, 16.50999999999999801, -5.016499999999999737 ) ) ;
#22427=DIRECTION ( 'NONE',  ( -0.000000000000000000, -0.000000000000000000, -1.000000000000000000 ) ) ;
#22442=CARTESIAN_POINT ( 'NONE',  ( 5.714078020757473730, 78.90256189635211115, -5.042866571093843397 ) ) ;
#22448=DIRECTION ( 'NONE',  ( 0.000000000000000000, 0.000000000000000000, 1.000000000000000000 ) ) ;
#22450=CYLINDRICAL_SURFACE ( 'NONE', #1675, 0.6350000000000001199 ) ;
#22475=CARTESIAN_POINT ( 'NONE',  ( 13.85159022459153988, 12.96416000000000146, -5.016499999999999737 ) ) ;
#22493=ORIENTED_EDGE ( 'NONE', *, *, #34761, .F. ) ;
#22498=CARTESIAN_POINT ( 'NONE',  ( -6.350000000000055600, 85.80437499999999318, 8.456951552361941263E-16 ) ) ;
#22509=EDGE_CURVE ( 'NONE', #19469, #296, #31252, .T. ) ;
#22524=CARTESIAN_POINT ( 'NONE',  ( -5.115874721081825172, 56.51499999999997215, -4.603382018214097648 ) ) ;
#22529=VERTEX_POINT ( 'NONE', #13147 ) ;
#22534=ORIENTED_EDGE ( 'NONE', *, *, #830, .T. ) ;
#22543=DIRECTION ( 'NONE',  ( -0.1469470846586743984, -9.335746474409589170E-17, 0.9891443546370349837 ) ) ;
#22547=DIRECTION ( 'NONE',  ( -0.7071067811865486830, -0.7071067811865464625, 8.659560562354946417E-17 ) ) ;
#22559=ORIENTED_EDGE ( 'NONE', *, *, #19654, .T. ) ;
#22572=VERTEX_POINT ( 'NONE', #36382 ) ;
#22573=CARTESIAN_POINT ( 'NONE',  ( 17.14499999999999957, 71.11999999999999034, -5.016499999999999737 ) ) ;
#22577=CARTESIAN_POINT ( 'NONE',  ( 10.92199999999999704, 12.96416000000000146, 0.000000000000000000 ) ) ;
#22580=VECTOR ( 'NONE', #21707, 1000.000000000000000 ) ;
#22600=CARTESIAN_POINT ( 'NONE',  ( 5.305748947172191698, 77.01756249999996840, 5.247078976224250013 ) ) ;
#22601=ORIENTED_EDGE ( 'NONE', *, *, #14115, .F. ) ;
#22617=ORIENTED_EDGE ( 'NONE', *, *, #10234, .F. ) ;
#22624=AXIS2_PLACEMENT_3D ( 'NONE', #9724, #41910, #25699 ) ;
#22638=CARTESIAN_POINT ( 'NONE',  ( -18.35410564743290962, 77.35382415001784295, -1.904999999999999583 ) ) ;
#22643=AXIS2_PLACEMENT_3D ( 'NONE', #25892, #31662, #38273 ) ;
#22648=VERTEX_POINT ( 'NONE', #35524 ) ;
#22653=CARTESIAN_POINT ( 'NONE',  ( 4.968812502025208744, 56.51947257897050036, -4.801689445572365322 ) ) ;
#22654=AXIS2_PLACEMENT_3D ( 'NONE', #16794, #23160, #19348 ) ;
#22657=DIRECTION ( 'NONE',  ( 0.000000000000000000, -1.000000000000000000, -0.000000000000000000 ) ) ;
#22660=DIRECTION ( 'NONE',  ( -6.353134868986659519E-16, 1.000000000000000000, 0.000000000000000000 ) ) ;
#22662=ORIENTED_EDGE ( 'NONE', *, *, #4319, .T. ) ;
#22672=CARTESIAN_POINT ( 'NONE',  ( 4.792324638247207780, 56.51998046905276141, 4.972049999977001811 ) ) ;
#22674=ORIENTED_EDGE ( 'NONE', *, *, #36852, .T. ) ;
#22679=EDGE_CURVE ( 'NONE', #25879, #27003, #6346, .T. ) ;
#22683=DIRECTION ( 'NONE',  ( -6.146657985744592735E-16, 3.905054717696928257E-31, 1.000000000000000000 ) ) ;
#22694=PRODUCT_DEFINITION_CONTEXT ( 'detailed design', #22944, 'design' ) ;
#22696=VERTEX_POINT ( 'NONE', #12723 ) ;
#22706=EDGE_CURVE ( 'NONE', #16646, #27187, #3363, .T. ) ;
#22711=EDGE_CURVE ( 'NONE', #40327, #35273, #39428, .T. ) ;
#22715=CARTESIAN_POINT ( 'NONE',  ( 5.354045385511907007, 57.14999999999996305, 5.213862164334982729 ) ) ;
#22720=VERTEX_POINT ( 'NONE', #42135 ) ;
#22726=CARTESIAN_POINT ( 'NONE',  ( 14.50851225146812595, 78.09971119798316863, 5.392902600000138769 ) ) ;
#22730=CARTESIAN_POINT ( 'NONE',  ( -4.966122758792669067, 56.51499999999997215, -4.710630977848821566 ) ) ;
#22737=CARTESIAN_POINT ( 'NONE',  ( -5.901202670473868928, 78.88741954747034413, -5.016800487701043920 ) ) ;
#22739=VERTEX_POINT ( 'NONE', #19524 ) ;
#22743=ADVANCED_FACE ( 'NONE', ( #6981, #26562 ), #32532, .T. ) ;
#22753=CARTESIAN_POINT ( 'NONE',  ( -13.85159022459153988, 16.50999999999999801, -5.016499999999999737 ) ) ;
#22768=VERTEX_POINT ( 'NONE', #20572 ) ;
#22785=DIRECTION ( 'NONE',  ( 9.627370216492862708E-17, 1.000000000000000000, -0.000000000000000000 ) ) ;
#22798=CARTESIAN_POINT ( 'NONE',  ( -10.92199999999999527, 55.98894877578615592, 6.098637220230963427E-16 ) ) ;
#22801=CARTESIAN_POINT ( 'NONE',  ( -6.059261036834082681, 78.87450423423038615, -5.016499999999999737 ) ) ;
#22805=EDGE_LOOP ( 'NONE', ( #14798, #20190, #39365, #6719, #20816, #32395, #10537, #33448, #15005, #11826 ) ) ;
#22806=CARTESIAN_POINT ( 'NONE',  ( 5.177913976931196594, 77.01756249999996840, 5.372100000000004094 ) ) ;
#22815=CARTESIAN_POINT ( 'NONE',  ( 6.059261036833978764, 78.87450423423040036, 5.016499999999999737 ) ) ;
#22817=CARTESIAN_POINT ( 'NONE',  ( 2.407412430484044816E-32, 1.626303258728256651E-15, 0.000000000000000000 ) ) ;
#22820=B_SPLINE_SURFACE_WITH_KNOTS ( 'NONE', 3, 1, ( 
 ( #6471, #19446 ),
 ( #2869, #3284 ),
 ( #15830, #29248 ),
 ( #92, #22834 ) ),
 .UNSPECIFIED., .F., .F., .F.,
 ( 4, 4 ),
 ( 2, 2 ),
 ( 0.000000000000000000, 0.6118630412642168670 ),
 ( 0.000000000000000000, 1.000000000000000000 ),
 .UNSPECIFIED. ) ;
#22826=EDGE_LOOP ( 'NONE', ( #36938, #11108, #13298, #11728, #2425, #15040, #5272 ) ) ;
#22830=VERTEX_POINT ( 'NONE', #33179 ) ;
#22834=CARTESIAN_POINT ( 'NONE',  ( 5.106395947886037234, 78.95054594174946772, -5.392902600000141433 ) ) ;
#22847=CARTESIAN_POINT ( 'NONE',  ( -5.871452009091383317, 65.30181249999996851, 5.016499999999999737 ) ) ;
#22864=CARTESIAN_POINT ( 'NONE',  ( 1.172031118611134874E-15, 12.17394877578616885, 0.000000000000000000 ) ) ;
#22870=CARTESIAN_POINT ( 'NONE',  ( -11.58677707360137532, 55.24499999999999034, 4.474811398758258285 ) ) ;
#22871=EDGE_CURVE ( 'NONE', #9633, #12494, #20994, .T. ) ;
#22872=CARTESIAN_POINT ( 'NONE',  ( 8.515285667870288113E-16, 8.844871939465425825, 0.000000000000000000 ) ) ;
#22885=VERTEX_POINT ( 'NONE', #27606 ) ;
#22908=AXIS2_PLACEMENT_3D ( 'NONE', #39763, #39972, #36764 ) ;
#22913=ADVANCED_FACE ( 'NONE', ( #26987 ), #33598, .T. ) ;
#22936=EDGE_CURVE ( 'NONE', #296, #31875, #30379, .T. ) ;
#22943=PLANE ( 'NONE',  #34920 ) ;
#22944=APPLICATION_CONTEXT ( 'automotive_design' ) ;
#22954=EDGE_LOOP ( 'NONE', ( #5622, #35866, #7879, #1166 ) ) ;
#22996=CARTESIAN_POINT ( 'NONE',  ( 18.35410564743290607, 77.35382415001784295, -1.904999999999999583 ) ) ;
#22997=CARTESIAN_POINT ( 'NONE',  ( 11.41714695485569564, 57.14999999999999858, 5.016499999999999737 ) ) ;
#22999=ADVANCED_FACE ( 'NONE', ( #4635 ), #10789, .F. ) ;
#23000=VECTOR ( 'NONE', #10402, 1000.000000000000114 ) ;
#23004=DIRECTION ( 'NONE',  ( -6.353134868986659519E-16, 1.000000000000000000, 0.000000000000000000 ) ) ;
#23021=ORIENTED_EDGE ( 'NONE', *, *, #12352, .T. ) ;
#23047=CARTESIAN_POINT ( 'NONE',  ( 6.349999999999945466, 86.35999999999998522, 0.000000000000000000 ) ) ;
#23054=FACE_OUTER_BOUND ( 'NONE', #36740, .T. ) ;
#23058=LINE ( 'NONE', #29474, #9864 ) ;
#23063=CARTESIAN_POINT ( 'NONE',  ( -6.059261036834474368, 65.30181249999996851, 5.016499999999999737 ) ) ;
#23064=CARTESIAN_POINT ( 'NONE',  ( -6.059261036834474368, 56.51499999999997925, 4.381499999999999950 ) ) ;
#23073=FACE_BOUND ( 'NONE', #7509, .T. ) ;
#23083=CARTESIAN_POINT ( 'NONE',  ( 6.059261036833978764, 78.87450423423040036, 5.016499999999999737 ) ) ;
#23084=FACE_OUTER_BOUND ( 'NONE', #38926, .T. ) ;
#23085=ORIENTED_EDGE ( 'NONE', *, *, #28433, .T. ) ;
#23087=ORIENTED_EDGE ( 'NONE', *, *, #39685, .F. ) ;
#23126=CARTESIAN_POINT ( 'NONE',  ( -14.24929227862422465, 61.25037559889041461, -5.016500000000000625 ) ) ;
#23140=CONICAL_SURFACE ( 'NONE', #4823, 14.73199999999999577, 0.7853981633974488341 ) ;
#23151=( BOUNDED_CURVE ( )  B_SPLINE_CURVE ( 3, ( #4053, #33436, #39831, #30013 ),
 .UNSPECIFIED., .F., .T. ) 
 B_SPLINE_CURVE_WITH_KNOTS ( ( 4, 4 ),
 ( 3.750906500318047510, 4.712388980384687898 ),
 .UNSPECIFIED. ) 
 CURVE ( )  GEOMETRIC_REPRESENTATION_ITEM ( )  RATIONAL_B_SPLINE_CURVE ( ( 1.000000000000000000, 0.9244349266169029633, 0.9244349266169029633, 1.000000000000000000 ) ) 
 REPRESENTATION_ITEM ( '' )  );
#23152=CARTESIAN_POINT ( 'NONE',  ( -5.354045385558898751, 56.51499999999976609, -5.213862164400199894 ) ) ;
#23160=DIRECTION ( 'NONE',  ( 0.000000000000000000, 1.000000000000000000, 0.000000000000000000 ) ) ;
#23161=B_SPLINE_SURFACE_WITH_KNOTS ( 'NONE', 5, 3, ( 
 ( #32220, #38413, #15595, #29010 ),
 ( #42029, #12621, #39240, #3470 ),
 ( #35415, #12825, #15803, #38821 ),
 ( #6659, #29439, #28811, #9225 ),
 ( #25813, #26024, #41827, #35213 ),
 ( #25609, #22600, #29222, #35631 ),
 ( #63, #9422, #13033, #39032 ),
 ( #9840, #22806, #35844, #3897 ) ),
 .UNSPECIFIED., .F., .F., .F.,
 ( 6, 2, 6 ),
 ( 4, 4 ),
 ( 0.000000000000000000, 0.5000000000000000000, 1.000000000000000000 ),
 ( -0.002373312499999995218, 0.03277393749999999578 ),
 .UNSPECIFIED. ) ;
#23166=CIRCLE ( 'NONE', #33398, 0.6350000000000001199 ) ;
#23170=CARTESIAN_POINT ( 'NONE',  ( -5.177913976931298734, 78.94499979771843812, -5.372100000000003206 ) ) ;
#23195=AXIS2_PLACEMENT_3D ( 'NONE', #30701, #17913, #2177 ) ;
#23199=ORIENTED_EDGE ( 'NONE', *, *, #677, .F. ) ;
#23202=VECTOR ( 'NONE', #30820, 1000.000000000000000 ) ;
#23218=CARTESIAN_POINT ( 'NONE',  ( -5.555120986090559931, 78.91530963298718859, 5.093895734005253750 ) ) ;
#23220=CARTESIAN_POINT ( 'NONE',  ( 17.14499999999999957, 71.11999999999999034, -5.016499999999999737 ) ) ;
#23232=ORIENTED_EDGE ( 'NONE', *, *, #35246, .T. ) ;
#23238=ADVANCED_FACE ( 'NONE', ( #28452 ), #2487, .F. ) ;
#23244=CARTESIAN_POINT ( 'NONE',  ( -6.350000000000036060, 57.78499999999998948, 7.776507174585692163E-16 ) ) ;
#23257=CIRCLE ( 'NONE', #14415, 2.540000000000000480 ) ;
#23265=AXIS2_PLACEMENT_3D ( 'NONE', #9203, #37962, #41379 ) ;
#23267=CARTESIAN_POINT ( 'NONE',  ( 5.177913976931196594, 78.94499979771845233, 5.372100000000001430 ) ) ;
#23272=LINE ( 'NONE', #29689, #20489 ) ;
#23274=CARTESIAN_POINT ( 'NONE',  ( -5.106395947886143816, 78.95054594174945350, -1.904999999999999583 ) ) ;
#23278=EDGE_CURVE ( 'NONE', #29922, #35053, #18808, .T. ) ;
#23294=CARTESIAN_POINT ( 'NONE',  ( -10.28897677580358305, 56.51499999999998636, 4.381500000000000838 ) ) ;
#23307=EDGE_CURVE ( 'NONE', #38115, #28439, #21067, .T. ) ;
#23309=EDGE_CURVE ( 'NONE', #20396, #5931, #2731, .T. ) ;
#23328=ORIENTED_EDGE ( 'NONE', *, *, #36023, .T. ) ;
#23332=ORIENTED_EDGE ( 'NONE', *, *, #17820, .F. ) ;
#23340=EDGE_LOOP ( 'NONE', ( #3832, #39362, #32720, #24175 ) ) ;
#23354=EDGE_CURVE ( 'NONE', #32592, #17039, #12708, .T. ) ;
#23362=ORIENTED_EDGE ( 'NONE', *, *, #25053, .T. ) ;
#23365=VECTOR ( 'NONE', #33718, 1000.000000000000000 ) ;
#23404=EDGE_CURVE ( 'NONE', #24559, #13560, #25478, .T. ) ;
#23417=CARTESIAN_POINT ( 'NONE',  ( 1.650612623617701257E-15, 17.14499999999999957, 0.000000000000000000 ) ) ;
#23421=DIRECTION ( 'NONE',  ( 1.000000000000000000, 6.353134868986659519E-16, 0.000000000000000000 ) ) ;
#23425=CARTESIAN_POINT ( 'NONE',  ( 14.39766717389552042, 12.96416000000000146, -1.904999999999999583 ) ) ;
#23432=CARTESIAN_POINT ( 'NONE',  ( -5.571852488405353299, 78.91397923090406152, 5.086862008547728742 ) ) ;
#23444=ORIENTED_EDGE ( 'NONE', *, *, #19844, .F. ) ;
#23465=ORIENTED_EDGE ( 'NONE', *, *, #22936, .F. ) ;
#23472=EDGE_CURVE ( 'NONE', #5073, #22768, #38883, .T. ) ;
#23477=EDGE_CURVE ( 'NONE', #16450, #4948, #41883, .T. ) ;
#23485=CARTESIAN_POINT ( 'NONE',  ( -5.353961914030953118, 56.51499999999979451, 5.213928161110560566 ) ) ;
#23518=DIRECTION ( 'NONE',  ( 5.463695987328526437E-16, -1.000000000000000000, -1.672774450599033775E-31 ) ) ;
#23522=CARTESIAN_POINT ( 'NONE',  ( -10.28897677580358305, 57.14999999999998437, 5.016499999999999737 ) ) ;
#23526=CARTESIAN_POINT ( 'NONE',  ( 13.85159022459153988, 57.78500000000000369, -5.016500000000005066 ) ) ;
#23530=ADVANCED_FACE ( 'NONE', ( #32703 ), #7117, .T. ) ;
#23538=ADVANCED_FACE ( 'NONE', ( #9485 ), #19273, .T. ) ;
#23543=EDGE_CURVE ( 'NONE', #9633, #12494, #26130, .T. ) ;
#23549=ORIENTED_EDGE ( 'NONE', *, *, #2134, .T. ) ;
#23569=ORIENTED_EDGE ( 'NONE', *, *, #23472, .T. ) ;
#23576=EDGE_LOOP ( 'NONE', ( #29447, #27060, #7134, #15338 ) ) ;
#23578=CARTESIAN_POINT ( 'NONE',  ( 13.85159022459153988, 59.63164443796365077, -5.016499999999999737 ) ) ;
#23586=DIRECTION ( 'NONE',  ( 0.9849462604886048966, 0.000000000000000000, -0.1728608224830406881 ) ) ;
#23613=CARTESIAN_POINT ( 'NONE',  ( 18.35410564743290607, 77.35382415001784295, -5.016499999999999737 ) ) ;
#23620=ORIENTED_EDGE ( 'NONE', *, *, #39798, .T. ) ;
#23633=VECTOR ( 'NONE', #21135, 1000.000000000000114 ) ;
#23637=CARTESIAN_POINT ( 'NONE',  ( 1.650612623617701651E-15, 17.14499999999999957, 0.000000000000000000 ) ) ;
#23642=CARTESIAN_POINT ( 'NONE',  ( 11.58677707360117282, 55.41127257906217807, 4.474811398756911807 ) ) ;
#23652=ADVANCED_FACE ( 'NONE', ( #23084 ), #35664, .T. ) ;
#23655=CARTESIAN_POINT ( 'NONE',  ( -5.249547377000530979, 56.51499999999963109, -4.563748390634326135 ) ) ;
#23656=B_SPLINE_CURVE_WITH_KNOTS ( 'NONE', 3,
 ( #26345, #19951, #29555, #1017 ),
 .UNSPECIFIED., .F., .F.,
 ( 4, 4 ),
 ( 0.000000000000000000, 0.5643836377221603806 ),
 .UNSPECIFIED. ) ;
#23679=ORIENTED_EDGE ( 'NONE', *, *, #30320, .F. ) ;
#23691=ADVANCED_FACE ( 'NONE', ( #38467 ), #22450, .T. ) ;
#23712=CIRCLE ( 'NONE', #34616, 2.540000000000000480 ) ;
#23720=CARTESIAN_POINT ( 'NONE',  ( -11.58677707360137532, 55.98894877578615592, 4.474811398758257397 ) ) ;
#23732=ADVANCED_FACE ( 'NONE', ( #42093 ), #12888, .F. ) ;
#23735=ORIENTED_EDGE ( 'NONE', *, *, #37593, .T. ) ;
#23750=CARTESIAN_POINT ( 'NONE',  ( 5.305748947172212127, 57.14999999999998437, 5.247078976224250013 ) ) ;
#23762=FACE_OUTER_BOUND ( 'NONE', #19118, .T. ) ;
#23767=DIRECTION ( 'NONE',  ( -1.000000000000000000, 9.627370216492862708E-17, 0.000000000000000000 ) ) ;
#23772=EDGE_CURVE ( 'NONE', #18200, #21005, #7352, .T. ) ;
#23782=B_SPLINE_CURVE_WITH_KNOTS ( 'NONE', 3,
 ( #12396, #25584, #16408, #9200, #25386, #32612, #38389, #34988 ),
 .UNSPECIFIED., .F., .F.,
 ( 4, 2, 2, 4 ),
 ( 0.003986743484052250597, 0.004242962777773736337, 0.004499182071495222077, 0.005011620658938190087 ),
 .UNSPECIFIED. ) ;
#23789=ORIENTED_EDGE ( 'NONE', *, *, #7400, .T. ) ;
#23807=ORIENTED_EDGE ( 'NONE', *, *, #25636, .F. ) ;
#23815=DIRECTION ( 'NONE',  ( -5.463695987328526437E-16, -1.000000000000000000, -1.672774450599033775E-31 ) ) ;
#23821=EDGE_CURVE ( 'NONE', #41231, #37437, #13735, .T. ) ;
#23859=CARTESIAN_POINT ( 'NONE',  ( 11.58677707360137354, 55.24500000000000455, 4.474811398758258285 ) ) ;
#23866=CARTESIAN_POINT ( 'NONE',  ( -5.177913976931298734, 78.94499979771843812, 5.372100000000002318 ) ) ;
#23871=CARTESIAN_POINT ( 'NONE',  ( -4.880629475887630520, 56.51998046905276141, -4.886937129208420494 ) ) ;
#23876=DIRECTION ( 'NONE',  ( 6.353134868986659519E-16, -1.000000000000000000, -0.000000000000000000 ) ) ;
#23896=EDGE_LOOP ( 'NONE', ( #8587, #10523 ) ) ;
#23899=CARTESIAN_POINT ( 'NONE',  ( 11.08653569745442091, 56.26057688450584493, -4.438844214435508029 ) ) ;
#23905=CIRCLE ( 'NONE', #6941, 18.13811525448111439 ) ;
#23912=LINE ( 'NONE', #11135, #33292 ) ;
#23913=DIRECTION ( 'NONE',  ( -6.353134868986659519E-16, 1.000000000000000000, 0.000000000000000000 ) ) ;
#23918=DIRECTION ( 'NONE',  ( 9.627370216492862708E-17, 1.000000000000000000, -0.000000000000000000 ) ) ;
#23932=DIRECTION ( 'NONE',  ( -6.353134868986659519E-16, 1.000000000000000000, -0.000000000000000000 ) ) ;
#23944=AXIS2_PLACEMENT_3D ( 'NONE', #8583, #31999, #2838 ) ;
#23947=CARTESIAN_POINT ( 'NONE',  ( -17.68910244842765778, 0.6350000000000018963, 2.166290269325653984E-15 ) ) ;
#23954=CARTESIAN_POINT ( 'NONE',  ( -4.792324638262704717, 56.51998046905272588, -4.972049999962482758 ) ) ;
#23957=VECTOR ( 'NONE', #17318, 999.9999999999998863 ) ;
#23963=CARTESIAN_POINT ( 'NONE',  ( -3.630816577625875226E-14, 57.14999999999999147, 0.000000000000000000 ) ) ;
#23992=EDGE_CURVE ( 'NONE', #6508, #18747, #30878, .T. ) ;
#24008=DIRECTION ( 'NONE',  ( 1.000000000000000000, -1.365923996832131856E-16, 0.000000000000000000 ) ) ;
#24019=ORIENTED_EDGE ( 'NONE', *, *, #38059, .T. ) ;
#24045=CIRCLE ( 'NONE', #5705, 0.6350000000000001199 ) ;
#24074=ORIENTED_EDGE ( 'NONE', *, *, #23543, .F. ) ;
#24080=DIRECTION ( 'NONE',  ( 6.353134868986659519E-16, -1.000000000000000000, 0.000000000000000000 ) ) ;
#24092=VECTOR ( 'NONE', #29074, 1000.000000000000114 ) ;
#24102=CARTESIAN_POINT ( 'NONE',  ( 6.984999999999963904, 57.14999999999999858, 8.554157892044261576E-16 ) ) ;
#24109=ORIENTED_EDGE ( 'NONE', *, *, #2466, .T. ) ;
#24111=CARTESIAN_POINT ( 'NONE',  ( 12.16475753114684011, 55.74362973025083079, -5.016500000000000625 ) ) ;
#24122=CARTESIAN_POINT ( 'NONE',  ( -20.83467972660109169, 65.95194780259438971, 5.016499999999999737 ) ) ;
#24133=ORIENTED_EDGE ( 'NONE', *, *, #1717, .F. ) ;
#24154=DIRECTION ( 'NONE',  ( -1.000000000000000000, 0.000000000000000000, 5.329070518200751394E-15 ) ) ;
#24155=( GEOMETRIC_REPRESENTATION_CONTEXT ( 3 ) GLOBAL_UNCERTAINTY_ASSIGNED_CONTEXT ( ( #38916 ) ) GLOBAL_UNIT_ASSIGNED_CONTEXT ( ( #19777, #32797, #35785 ) ) REPRESENTATION_CONTEXT ( 'NONE', 'WORKASPACE' ) );
#24159=CARTESIAN_POINT ( 'NONE',  ( 10.92199999999999704, 17.14499999999999957, -5.850485014536587995E-17 ) ) ;
#24175=ORIENTED_EDGE ( 'NONE', *, *, #22711, .T. ) ;
#24184=CARTESIAN_POINT ( 'NONE',  ( 5.565035070531680006, 78.91452218770625393, -5.089667964246464393 ) ) ;
#24212=CARTESIAN_POINT ( 'NONE',  ( 10.92199999999999704, 56.51500000000000057, -4.381499999999999950 ) ) ;
#24216=DIRECTION ( 'NONE',  ( 1.000000000000000000, 0.000000000000000000, 0.000000000000000000 ) ) ;
#24223=EDGE_CURVE ( 'NONE', #11069, #34925, #40442, .T. ) ;
#24253=VERTEX_POINT ( 'NONE', #17888 ) ;
#24258=VERTEX_POINT ( 'NONE', #40702 ) ;
#24259=AXIS2_PLACEMENT_3D ( 'NONE', #19386, #18968, #31975 ) ;
#24269=CARTESIAN_POINT ( 'NONE',  ( 16.87828382557106721, 17.14499999999999957, 5.016499999999999737 ) ) ;
#24274=CARTESIAN_POINT ( 'NONE',  ( 1.650612623617701257E-15, 17.14499999999999957, 0.000000000000000000 ) ) ;
#24288=FACE_OUTER_BOUND ( 'NONE', #20144, .T. ) ;
#24301=ORIENTED_EDGE ( 'NONE', *, *, #19302, .F. ) ;
#24303=CIRCLE ( 'NONE', #14024, 6.349999999999999645 ) ;
#24317=EDGE_CURVE ( 'NONE', #35912, #449, #16172, .T. ) ;
#24328=CARTESIAN_POINT ( 'NONE',  ( -10.94257363143063166, 56.35470871607765275, 4.428493390990959178 ) ) ;
#24337=DIRECTION ( 'NONE',  ( -0.000000000000000000, -0.000000000000000000, -1.000000000000000000 ) ) ;
#24339=CARTESIAN_POINT ( 'NONE',  ( 5.177913976931217910, 56.99702125087949156, -5.372099999999997877 ) ) ;
#24345=CARTESIAN_POINT ( 'NONE',  ( 11.66725022231030984, 17.14499999999999957, 5.016499999999999737 ) ) ;
#24356=CARTESIAN_POINT ( 'NONE',  ( 6.059261036834406866, 57.14999999999999858, 5.016499999999999737 ) ) ;
#24367=ADVANCED_FACE ( 'NONE', ( #29151 ), #12351, .T. ) ;
#24379=VECTOR ( 'NONE', #39015, 1000.000000000000000 ) ;
#24388=ORIENTED_EDGE ( 'NONE', *, *, #33723, .F. ) ;
#24410=ORIENTED_EDGE ( 'NONE', *, *, #25627, .T. ) ;
#24425=CARTESIAN_POINT ( 'NONE',  ( -9.665786669610962889, 55.24499999999999034, -0.1866227975165204167 ) ) ;
#24436=AXIS2_PLACEMENT_3D ( 'NONE', #17278, #11303, #7496 ) ;
#24451=CARTESIAN_POINT ( 'NONE',  ( 5.177913976931196594, 77.01756249999996840, -5.372100000000004094 ) ) ;
#24463=ORIENTED_EDGE ( 'NONE', *, *, #26125, .F. ) ;
#24478=CARTESIAN_POINT ( 'NONE',  ( 10.62867326514804311, 56.48194529650096740, 4.405924061720294382 ) ) ;
#24479=CARTESIAN_POINT ( 'NONE',  ( -6.059261036834473479, 56.58343591620776181, -4.712961528314683513 ) ) ;
#24494=ADVANCED_FACE ( 'NONE', ( #9775 ), #32787, .F. ) ;
#24504=ORIENTED_EDGE ( 'NONE', *, *, #16439, .F. ) ;
#24513=LINE ( 'NONE', #11957, #33139 ) ;
#24541=CARTESIAN_POINT ( 'NONE',  ( 18.35410564743290607, 77.35382415001784295, -1.904999999999999583 ) ) ;
#24550=VECTOR ( 'NONE', #4294, 1000.000000000000000 ) ;
#24559=VERTEX_POINT ( 'NONE', #17112 ) ;
#24568=ORIENTED_EDGE ( 'NONE', *, *, #1463, .T. ) ;
#24572=TOROIDAL_SURFACE ( 'NONE', #1466, 6.826249999999999929, 0.6350000000000000089 ) ;
#24581=EDGE_CURVE ( 'NONE', #4948, #20977, #40139, .T. ) ;
#24583=VERTEX_POINT ( 'NONE', #30314 ) ;
#24598=VECTOR ( 'NONE', #24652, 1000.000000000000000 ) ;
#24625=DIRECTION ( 'NONE',  ( 9.627370216492862708E-17, 1.000000000000000000, -0.000000000000000000 ) ) ;
#24631=VECTOR ( 'NONE', #15114, 1000.000000000000227 ) ;
#24642=AXIS2_PLACEMENT_3D ( 'NONE', #7997, #11384, #37173 ) ;
#24644=ORIENTED_EDGE ( 'NONE', *, *, #5173, .F. ) ;
#24652=DIRECTION ( 'NONE',  ( -1.000000000000000000, -6.353134868986659519E-16, 0.000000000000000000 ) ) ;
#24676=ORIENTED_EDGE ( 'NONE', *, *, #15903, .F. ) ;
#24686=CARTESIAN_POINT ( 'NONE',  ( -5.177913976931285411, 57.14999999999998437, 5.372100000000002318 ) ) ;
#24692=VECTOR ( 'NONE', #3259, 1000.000000000000000 ) ;
#24698=ORIENTED_EDGE ( 'NONE', *, *, #29088, .F. ) ;
#24707=DIRECTION ( 'NONE',  ( 9.627370216492862708E-17, 1.000000000000000000, -0.000000000000000000 ) ) ;
#24708=CARTESIAN_POINT ( 'NONE',  ( -14.81953868692883702, 57.78499999999998948, 0.4987879908248463168 ) ) ;
#24712=DIRECTION ( 'NONE',  ( -1.000000000000000000, 0.000000000000000000, 0.000000000000000000 ) ) ;
#24717=ORIENTED_EDGE ( 'NONE', *, *, #41947, .F. ) ;
#24735=FACE_OUTER_BOUND ( 'NONE', #20868, .T. ) ;
#24762=ADVANCED_FACE ( 'NONE', ( #33010 ), #16155, .F. ) ;
#24777=ORIENTED_EDGE ( 'NONE', *, *, #22679, .F. ) ;
#24805=CARTESIAN_POINT ( 'NONE',  ( -16.62722885652246418, 62.94807988814252298, 4.514343177587269551 ) ) ;
#24819=CARTESIAN_POINT ( 'NONE',  ( 10.28897677580358305, 56.51500000000000057, -4.381500000000000838 ) ) ;
#24827=VERTEX_POINT ( 'NONE', #12302 ) ;
#24839=EDGE_CURVE ( 'NONE', #31005, #5931, #18252, .T. ) ;
#24843=CARTESIAN_POINT ( 'NONE',  ( 13.51778232847667205, 17.08230797367789222, -5.016499999999999737 ) ) ;
#24859=CARTESIAN_POINT ( 'NONE',  ( 5.449044798800651179, 56.51500000000380197, -5.145813327034902684 ) ) ;
#24906=CARTESIAN_POINT ( 'NONE',  ( 6.059261036834406866, 57.14999999999999858, -5.016499999999999737 ) ) ;
#24908=CARTESIAN_POINT ( 'NONE',  ( 10.28897677580357950, 57.14999999999999858, 5.016499999999999737 ) ) ;
#24909=CARTESIAN_POINT ( 'NONE',  ( -14.91798719394653538, 12.51401280605346145, 2.024102502787695046E-15 ) ) ;
#24912=VECTOR ( 'NONE', #12661, 1000.000000000000000 ) ;
#24940=VERTEX_POINT ( 'NONE', #8267 ) ;
#24950=CARTESIAN_POINT ( 'NONE',  ( -5.309060684617390516E-14, 83.56599999999998829, 0.000000000000000000 ) ) ;
#24957=CARTESIAN_POINT ( 'NONE',  ( -14.94465077092626970, 61.74681991364688827, 5.072843609925764774 ) ) ;
#24971=CARTESIAN_POINT ( 'NONE',  ( -6.059261036834082681, 78.87450423423038615, -5.016499999999999737 ) ) ;
#25005=EDGE_CURVE ( 'NONE', #21058, #37417, #30154, .T. ) ;
#25008=CARTESIAN_POINT ( 'NONE',  ( 6.059261036834389103, 56.51500000000000057, 4.381499999999999950 ) ) ;
#25013=CARTESIAN_POINT ( 'NONE',  ( 14.73199999999999754, 61.59499999999999886, -5.016499999999999737 ) ) ;
#25016=CARTESIAN_POINT ( 'NONE',  ( -6.057513928997650510, 83.56599999999998829, -1.904999999999999805 ) ) ;
#25018=CARTESIAN_POINT ( 'NONE',  ( -5.305748947172302721, 88.73331249999999670, -5.247078976224250013 ) ) ;
#25021=ORIENTED_EDGE ( 'NONE', *, *, #5067, .F. ) ;
#25024=CARTESIAN_POINT ( 'NONE',  ( 16.87828382557106721, 17.14499999999999957, 0.000000000000000000 ) ) ;
#25030=CARTESIAN_POINT ( 'NONE',  ( 5.385891243465063205, 78.92849802251100755, -5.190125708699709683 ) ) ;
#25033=DIRECTION ( 'NONE',  ( -0.000000000000000000, -0.000000000000000000, -1.000000000000000000 ) ) ;
#25041=LINE ( 'NONE', #8864, #19757 ) ;
#25053=EDGE_CURVE ( 'NONE', #22768, #6508, #32193, .T. ) ;
#25063=FACE_OUTER_BOUND ( 'NONE', #30449, .T. ) ;
#25083=FACE_OUTER_BOUND ( 'NONE', #2804, .T. ) ;
#25084=CARTESIAN_POINT ( 'NONE',  ( 6.262914499211069241, 78.85772796343783853, -4.069400916056300055 ) ) ;
#25085=CARTESIAN_POINT ( 'NONE',  ( -23.49500000000000455, 71.11999999999999034, -1.904999999999999583 ) ) ;
#25100=ORIENTED_EDGE ( 'NONE', *, *, #7471, .T. ) ;
#25114=CARTESIAN_POINT ( 'NONE',  ( 5.348924234570989533, 56.51499999999999346, 4.492130288940735738 ) ) ;
#25117=VECTOR ( 'NONE', #5504, 1000.000000000000114 ) ;
#25118=AXIS2_PLACEMENT_3D ( 'NONE', #26821, #23815, #20612 ) ;
#25128=ORIENTED_EDGE ( 'NONE', *, *, #31380, .T. ) ;
#25141=CARTESIAN_POINT ( 'NONE',  ( -5.348924234571056147, 56.51499999999999346, 4.492130288940740179 ) ) ;
#25146=ORIENTED_EDGE ( 'NONE', *, *, #6109, .T. ) ;
#25156=VERTEX_POINT ( 'NONE', #22281 ) ;
#25162=AXIS2_PLACEMENT_3D ( 'NONE', #33382, #26777, #29965 ) ;
#25167=DIRECTION ( 'NONE',  ( 0.000000000000000000, 0.000000000000000000, 1.000000000000000000 ) ) ;
#25171=ORIENTED_EDGE ( 'NONE', *, *, #7929, .F. ) ;
#25173=CARTESIAN_POINT ( 'NONE',  ( 10.28897677580358128, 56.51500000000000057, 4.381499999999999950 ) ) ;
#25174=DIRECTION ( 'NONE',  ( 0.1715592850456333363, -0.1224830539174543431, 0.9775302108976914317 ) ) ;
#25194=CARTESIAN_POINT ( 'NONE',  ( -9.665786669610962889, 56.51499999999998636, 0.1866227975165156705 ) ) ;
#25206=LINE ( 'NONE', #29234, #15886 ) ;
#25213=B_SPLINE_CURVE_WITH_KNOTS ( 'NONE', 3,
 ( #26446, #12819, #3891, #22801 ),
 .UNSPECIFIED., .F., .F.,
 ( 4, 4 ),
 ( 0.000000000000000000, 0.5643836377221552736 ),
 .UNSPECIFIED. ) ;
#25235=CARTESIAN_POINT ( 'NONE',  ( -5.177913976931283635, 53.58606249999999704, -5.372100000000000541 ) ) ;
#25239=ORIENTED_EDGE ( 'NONE', *, *, #10766, .F. ) ;
#25269=CARTESIAN_POINT ( 'NONE',  ( -2.032601633563780229E-14, 30.83083951148100255, -1.904999999999999805 ) ) ;
#25279=CARTESIAN_POINT ( 'NONE',  ( 5.860205464924936436, 57.15000000000087255, -5.019550311879306115 ) ) ;
#25280=CIRCLE ( 'NONE', #27323, 6.349999999999999645 ) ;
#25285=CARTESIAN_POINT ( 'NONE',  ( -5.941750549330245157, 56.51500000000488200, 5.016499812855502505 ) ) ;
#25289=CARTESIAN_POINT ( 'NONE',  ( -17.14499999999999957, 71.11999999999999034, -5.016499999999999737 ) ) ;
#25294=ORIENTED_EDGE ( 'NONE', *, *, #7649, .F. ) ;
#25304=DIRECTION ( 'NONE',  ( -0.8138664877804109299, 0.5810519254489895369, 0.000000000000000000 ) ) ;
#25311=EDGE_CURVE ( 'NONE', #26988, #20298, #14470, .T. ) ;
#25317=AXIS2_PLACEMENT_3D ( 'NONE', #26230, #3251, #19830 ) ;
#25329=EDGE_CURVE ( 'NONE', #25936, #31634, #41636, .T. ) ;
#25349=CARTESIAN_POINT ( 'NONE',  ( 17.14499999999999957, 71.11999999999999034, 5.016499999999999737 ) ) ;
#25354=DIRECTION ( 'NONE',  ( -1.000000000000000000, 0.000000000000000000, 0.000000000000000000 ) ) ;
#25364=VERTEX_POINT ( 'NONE', #12925 ) ;
#25365=ORIENTED_EDGE ( 'NONE', *, *, #41005, .F. ) ;
#25374=DIRECTION ( 'NONE',  ( -0.000000000000000000, -0.000000000000000000, -1.000000000000000000 ) ) ;
#25386=CARTESIAN_POINT ( 'NONE',  ( -13.70915846191426013, 16.90875728684043366, 5.016499999999999737 ) ) ;
#25393=AXIS2_PLACEMENT_3D ( 'NONE', #24425, #40850, #5290 ) ;
#25402=EDGE_CURVE ( 'NONE', #37685, #4530, #39518, .T. ) ;
#25420=CONICAL_SURFACE ( 'NONE', #22643, 13.46199999999999619, 0.7853981633974497223 ) ;
#25452=CARTESIAN_POINT ( 'NONE',  ( -5.475330206976867231, 53.58606249999999704, -5.107412922131463695 ) ) ;
#25455=ORIENTED_EDGE ( 'NONE', *, *, #37587, .T. ) ;
#25465=CARTESIAN_POINT ( 'NONE',  ( 5.767947771861689610, 78.89823565723094134, -5.032924692340810857 ) ) ;
#25468=DIRECTION ( 'NONE',  ( 2.664535259100375303E-15, 0.000000000000000000, 1.000000000000000000 ) ) ;
#25472=DIRECTION ( 'NONE',  ( -9.627370216492862708E-17, -1.000000000000000000, 0.000000000000000000 ) ) ;
#25473=ORIENTED_EDGE ( 'NONE', *, *, #4045, .T. ) ;
#25478=CIRCLE ( 'NONE', #15899, 14.73199999999999577 ) ;
#25497=PLANE ( 'NONE',  #27653 ) ;
#25503=CARTESIAN_POINT ( 'NONE',  ( 13.85159022459154166, 60.48513866567135722, 5.016500000000000625 ) ) ;
#25509=CARTESIAN_POINT ( 'NONE',  ( 17.14499999999999957, 71.11999999999999034, 1.904999999999989146 ) ) ;
#25510=CARTESIAN_POINT ( 'NONE',  ( 1.406077420118782567E-15, 14.60500000000000220, 0.000000000000000000 ) ) ;
#25515=CARTESIAN_POINT ( 'NONE',  ( 5.224239234539634680, 57.14999999999999147, 5.327449267724802873 ) ) ;
#25530=DIRECTION ( 'NONE',  ( 1.000000000000000000, -9.466894658874049451E-17, 0.000000000000000000 ) ) ;
#25533=ADVANCED_FACE ( 'NONE', ( #23762 ), #1427, .F. ) ;
#25543=ORIENTED_EDGE ( 'NONE', *, *, #30098, .F. ) ;
#25551=DIRECTION ( 'NONE',  ( -1.000000000000000000, 5.463695987328526437E-16, -6.146657985744592735E-16 ) ) ;
#25560=VERTEX_POINT ( 'NONE', #13566 ) ;
#25582=LINE ( 'NONE', #39427, #4106 ) ;
#25584=CARTESIAN_POINT ( 'NONE',  ( -13.85159022459154166, 16.59642619247577500, 5.016500000000000625 ) ) ;
#25588=DIRECTION ( 'NONE',  ( 1.000000000000000000, 0.000000000000000000, 0.000000000000000000 ) ) ;
#25591=LINE ( 'NONE', #46, #40739 ) ;
#25598=DIRECTION ( 'NONE',  ( -6.353134868986659519E-16, 1.000000000000000000, 0.000000000000000000 ) ) ;
#25602=DIRECTION ( 'NONE',  ( 9.627370216492862708E-17, 1.000000000000000000, -0.000000000000000000 ) ) ;
#25603=DIRECTION ( 'NONE',  ( 0.000000000000000000, 1.000000000000000000, 0.000000000000000000 ) ) ;
#25608=ADVANCED_FACE ( 'NONE', ( #39990 ), #20563, .T. ) ;
#25609=CARTESIAN_POINT ( 'NONE',  ( 5.305748947172191698, 88.73331249999999670, 5.247078976224250013 ) ) ;
#25627=EDGE_CURVE ( 'NONE', #18019, #7919, #36304, .T. ) ;
#25636=EDGE_CURVE ( 'NONE', #5073, #19034, #19289, .T. ) ;
#25639=FACE_BOUND ( 'NONE', #17385, .T. ) ;
#25643=DIRECTION ( 'NONE',  ( 1.000000000000000000, 6.353134868986659519E-16, 0.000000000000000000 ) ) ;
#25651=CARTESIAN_POINT ( 'NONE',  ( -6.059261036834474368, 53.58606249999999704, -5.016499999999999737 ) ) ;
#25664=CARTESIAN_POINT ( 'NONE',  ( 5.800481910058622681, 78.89561208401062231, -5.028344476440722133 ) ) ;
#25668=DIRECTION ( 'NONE',  ( -0.000000000000000000, -1.000000000000000000, -0.000000000000000000 ) ) ;
#25682=EDGE_CURVE ( 'NONE', #33118, #24559, #1638, .T. ) ;
#25693=CARTESIAN_POINT ( 'NONE',  ( -17.14499999999999957, 71.11999999999999034, 1.904999999999989146 ) ) ;
#25699=DIRECTION ( 'NONE',  ( 0.000000000000000000, 0.000000000000000000, -1.000000000000000000 ) ) ;
#25703=VERTEX_POINT ( 'NONE', #24819 ) ;
#25719=CARTESIAN_POINT ( 'NONE',  ( -6.059261036834082681, 78.87450423423038615, 5.016499999999999737 ) ) ;
#25727=DIRECTION ( 'NONE',  ( 6.353134868986659519E-16, -1.000000000000000000, -0.000000000000000000 ) ) ;
#25730=ORIENTED_EDGE ( 'NONE', *, *, #25005, .T. ) ;
#25733=CARTESIAN_POINT ( 'NONE',  ( 19.68500000000000227, 71.11999999999999034, 5.016499999999999737 ) ) ;
#25737=CARTESIAN_POINT ( 'NONE',  ( 12.21488373879589417, 55.24500000000000455, -5.016499999999999737 ) ) ;
#25738=CARTESIAN_POINT ( 'NONE',  ( -6.057513928997659391, 86.35999999999998522, -1.904999999999999805 ) ) ;
#25739=CARTESIAN_POINT ( 'NONE',  ( 5.177913976931196594, 78.94499979771845233, 5.372100000000001430 ) ) ;
#25746=VERTEX_POINT ( 'NONE', #34418 ) ;
#25756=CARTESIAN_POINT ( 'NONE',  ( -6.059261036834475256, 56.81853847168529370, 4.948064083792229617 ) ) ;
#25762=CARTESIAN_POINT ( 'NONE',  ( -12.21488373879589240, 17.14500000000000313, -4.381499999999999950 ) ) ;
#25773=DIRECTION ( 'NONE',  ( 0.8138664877804110409, -0.5810519254489896479, 5.002558946445370251E-16 ) ) ;
#25787=AXIS2_PLACEMENT_3D ( 'NONE', #10673, #29854, #10883 ) ;
#25812=ORIENTED_EDGE ( 'NONE', *, *, #36768, .F. ) ;
#25813=CARTESIAN_POINT ( 'NONE',  ( 5.475330206976777525, 88.73331249999999670, 5.107412922131463695 ) ) ;
#25814=AXIS2_PLACEMENT_3D ( 'NONE', #16546, #39353, #19952 ) ;
#25852=LINE ( 'NONE', #32679, #3908 ) ;
#25854=FACE_OUTER_BOUND ( 'NONE', #13203, .T. ) ;
#25872=DIRECTION ( 'NONE',  ( 0.000000000000000000, 0.000000000000000000, 1.000000000000000000 ) ) ;
#25876=DIRECTION ( 'NONE',  ( -0.8138664877804109299, -0.5810519254489895369, 0.000000000000000000 ) ) ;
#25879=VERTEX_POINT ( 'NONE', #31206 ) ;
#25892=CARTESIAN_POINT ( 'NONE',  ( 1.172031118611134874E-15, 12.17394877578616885, 0.000000000000000000 ) ) ;
#25893=CIRCLE ( 'NONE', #31338, 2.540000000000000480 ) ;
#25896=ORIENTED_EDGE ( 'NONE', *, *, #15368, .T. ) ;
#25907=DIRECTION ( 'NONE',  ( 0.000000000000000000, 1.000000000000000000, 0.000000000000000000 ) ) ;
#25909=EDGE_CURVE ( 'NONE', #29922, #33599, #31884, .T. ) ;
#25922=DIRECTION ( 'NONE',  ( 9.627370216492862708E-17, 1.000000000000000000, -0.000000000000000000 ) ) ;
#25932=EDGE_LOOP ( 'NONE', ( #28642, #6084 ) ) ;
#25936=VERTEX_POINT ( 'NONE', #31849 ) ;
#25940=AXIS2_PLACEMENT_3D ( 'NONE', #28737, #40903, #21908 ) ;
#25945=FACE_OUTER_BOUND ( 'NONE', #27515, .T. ) ;
#25956=ORIENTED_EDGE ( 'NONE', *, *, #14101, .T. ) ;
#25958=DIRECTION ( 'NONE',  ( -0.000000000000000000, -0.000000000000000000, -1.000000000000000000 ) ) ;
#25962=DIRECTION ( 'NONE',  ( -1.000000000000000000, 0.000000000000000000, 0.000000000000000000 ) ) ;
#25975=ORIENTED_EDGE ( 'NONE', *, *, #38073, .F. ) ;
#26000=DIRECTION ( 'NONE',  ( -0.1728608224830406603, -0.000000000000000000, -0.9849462604886047856 ) ) ;
#26003=VECTOR ( 'NONE', #2583, 1000.000000000000000 ) ;
#26004=DIRECTION ( 'NONE',  ( -9.627370216492862708E-17, -1.000000000000000000, 0.000000000000000000 ) ) ;
#26017=CARTESIAN_POINT ( 'NONE',  ( -15.50061618130080987, 62.14374591690594940, 1.904999999999990035 ) ) ;
#26018=DIRECTION ( 'NONE',  ( 2.664535259100375697E-15, 0.000000000000000000, 1.000000000000000000 ) ) ;
#26024=CARTESIAN_POINT ( 'NONE',  ( 5.475330206976777525, 77.01756249999996840, 5.107412922131463695 ) ) ;
#26044=ORIENTED_EDGE ( 'NONE', *, *, #37027, .F. ) ;
#26054=EDGE_CURVE ( 'NONE', #15866, #4432, #37462, .T. ) ;
#26057=CARTESIAN_POINT ( 'NONE',  ( -5.451267667241070720E-14, 85.80437499999999318, 0.000000000000000000 ) ) ;
#26065=CARTESIAN_POINT ( 'NONE',  ( -5.305748947172302721, 77.01756250000002524, 5.247078976224250013 ) ) ;
#26066=CARTESIAN_POINT ( 'NONE',  ( -5.941750550382311147, 57.15000000000365077, 5.016500000000000625 ) ) ;
#26076=ORIENTED_EDGE ( 'NONE', *, *, #13555, .T. ) ;
#26082=AXIS2_PLACEMENT_3D ( 'NONE', #15210, #12022, #34613 ) ;
#26088=DIRECTION ( 'NONE',  ( -0.000000000000000000, -1.000000000000000000, -0.000000000000000000 ) ) ;
#26089=DIRECTION ( 'NONE',  ( -6.353134868986659519E-16, 1.000000000000000000, 0.000000000000000000 ) ) ;
#26092=ORIENTED_EDGE ( 'NONE', *, *, #16981, .T. ) ;
#26093=ADVANCED_FACE ( 'NONE', ( #35687 ), #11807, .F. ) ;
#26094=CARTESIAN_POINT ( 'NONE',  ( 14.95453923199683111, 61.75387968257833649, 5.016499999999999737 ) ) ;
#26115=CARTESIAN_POINT ( 'NONE',  ( -6.059261036834472591, 57.14999999999998437, 5.016499999999999737 ) ) ;
#26125=EDGE_CURVE ( 'NONE', #39961, #11997, #41989, .T. ) ;
#26130=CIRCLE ( 'NONE', #14568, 14.73199999999999577 ) ;
#26139=DIRECTION ( 'NONE',  ( 6.353134868986659519E-16, -1.000000000000000000, 0.000000000000000000 ) ) ;
#26145=CARTESIAN_POINT ( 'NONE',  ( 4.966122758792402614, 56.51499999999995083, 4.710630977848971668 ) ) ;
#26158=CARTESIAN_POINT ( 'NONE',  ( 9.094996104468812348, 78.64197151092923832, 5.392902600000138769 ) ) ;
#26177=CARTESIAN_POINT ( 'NONE',  ( -6.059261036834476144, 56.51499999999998636, 4.381499999999999950 ) ) ;
#26181=PRESENTATION_STYLE_ASSIGNMENT (( #3628 ) ) ;
#26182=CARTESIAN_POINT ( 'NONE',  ( -6.905625000000052971, 85.80437499999999318, 8.456951552361939290E-16 ) ) ;
#26212=LINE ( 'NONE', #6421, #19115 ) ;
#26230=CARTESIAN_POINT ( 'NONE',  ( 8.947566919452587848E-16, 9.293884745518887769, 0.000000000000000000 ) ) ;
#26235=FACE_OUTER_BOUND ( 'NONE', #31587, .T. ) ;
#26246=B_SPLINE_SURFACE_WITH_KNOTS ( 'NONE', 5, 3, ( 
 ( #7456, #24451, #20835, #30019 ),
 ( #11461, #30228, #14239, #37055 ),
 ( #4478, #30646, #26830, #27245 ),
 ( #30854, #17853, #1067, #40261 ),
 ( #13832, #7873, #37455, #37254 ),
 ( #14035, #7665, #27456, #27039 ),
 ( #859, #40048, #1489, #40669 ),
 ( #40469, #11260, #20413, #33859 ) ),
 .UNSPECIFIED., .F., .F., .F.,
 ( 6, 2, 6 ),
 ( 4, 4 ),
 ( 0.000000000000000000, 0.5000000000000000000, 1.000000000000000000 ),
 ( -0.002373312499999995218, 0.03277393749999999578 ),
 .UNSPECIFIED. ) ;
#26256=ORIENTED_EDGE ( 'NONE', *, *, #41215, .F. ) ;
#26268=ORIENTED_EDGE ( 'NONE', *, *, #2518, .T. ) ;
#26274=CARTESIAN_POINT ( 'NONE',  ( -5.965356522962928842, 53.58606250000000415, 5.016499999999999737 ) ) ;
#26298=VERTEX_POINT ( 'NONE', #7663 ) ;
#26319=VECTOR ( 'NONE', #22173, 1000.000000000000000 ) ;
#26320=ORIENTED_EDGE ( 'NONE', *, *, #37367, .T. ) ;
#26322=CARTESIAN_POINT ( 'NONE',  ( -5.309060684617390516E-14, 83.56599999999998829, 0.000000000000000000 ) ) ;
#26333=ORIENTED_EDGE ( 'NONE', *, *, #9706, .F. ) ;
#26345=CARTESIAN_POINT ( 'NONE',  ( 18.35410564743290607, 77.35382415001784295, 5.016499999999999737 ) ) ;
#26358=CARTESIAN_POINT ( 'NONE',  ( 7.461249999999945537, 86.35999999999998522, 0.000000000000000000 ) ) ;
#26364=ORIENTED_EDGE ( 'NONE', *, *, #41193, .T. ) ;
#26367=CARTESIAN_POINT ( 'NONE',  ( -6.057513928997641628, 57.78499999999998948, -1.904999999999999805 ) ) ;
#26372=CARTESIAN_POINT ( 'NONE',  ( -5.224085778414857550, 56.51500000000001478, -4.542437760755098530 ) ) ;
#26401=CARTESIAN_POINT ( 'NONE',  ( -3.671158984043940170E-14, 57.78499999999999659, 0.000000000000000000 ) ) ;
#26409=ORIENTED_EDGE ( 'NONE', *, *, #40491, .T. ) ;
#26425=CARTESIAN_POINT ( 'NONE',  ( -10.92199999999999704, 16.51000000000000156, 0.000000000000000000 ) ) ;
#26429=AXIS2_PLACEMENT_3D ( 'NONE', #19662, #39071, #39280 ) ;
#26433=LINE ( 'NONE', #23425, #39906 ) ;
#26441=CARTESIAN_POINT ( 'NONE',  ( -10.28897677580358128, 56.51499999999998636, -4.381499999999999950 ) ) ;
#26446=CARTESIAN_POINT ( 'NONE',  ( -18.35410564743290607, 77.35382415001784295, -5.016499999999999737 ) ) ;
#26451=FACE_OUTER_BOUND ( 'NONE', #35727, .T. ) ;
#26453=CARTESIAN_POINT ( 'NONE',  ( -5.460438898883190006, 56.51499999999997215, 4.448267477574868067 ) ) ;
#26486=AXIS2_PLACEMENT_3D ( 'NONE', #26182, #33228, #35577 ) ;
#26493=CARTESIAN_POINT ( 'NONE',  ( -5.305748947172281405, 53.58606250000000415, 5.247078976224250013 ) ) ;
#26514=CARTESIAN_POINT ( 'NONE',  ( -10.86251533436417915, 78.45482716897161879, -1.904999999999999583 ) ) ;
#26532=AXIS2_PLACEMENT_3D ( 'NONE', #5259, #12264, #21197 ) ;
#26561=CARTESIAN_POINT ( 'NONE',  ( -6.059261036834475256, 57.15000000000000568, 5.016499999999999737 ) ) ;
#26562=FACE_BOUND ( 'NONE', #5748, .T. ) ;
#26579=CARTESIAN_POINT ( 'NONE',  ( -5.106395947886140263, 78.95054594174945350, 5.392902600000138769 ) ) ;
#26586=CARTESIAN_POINT ( 'NONE',  ( 10.28897677580358305, 57.14999999999999858, -5.016499999999999737 ) ) ;
#26593=EDGE_CURVE ( 'NONE', #36287, #22648, #8700, .T. ) ;
#26595=DIRECTION ( 'NONE',  ( 0.000000000000000000, 0.000000000000000000, 1.000000000000000000 ) ) ;
#26638=CARTESIAN_POINT ( 'NONE',  ( 11.58677707360137710, 55.24500000000000455, -4.474811398758258285 ) ) ;
#26643=CARTESIAN_POINT ( 'NONE',  ( 11.32678463655034129, 56.02547433970789115, 4.456118031212549013 ) ) ;
#26651=AXIS2_PLACEMENT_3D ( 'NONE', #18505, #31510, #2357 ) ;
#26670=CARTESIAN_POINT ( 'NONE',  ( 5.981046608238687057, 78.88093534801383555, 5.016500000000000625 ) ) ;
#26677=( BOUNDED_CURVE ( )  B_SPLINE_CURVE ( 3, ( #3388, #16354, #19136, #3607 ),
 .UNSPECIFIED., .F., .T. ) 
 B_SPLINE_CURVE_WITH_KNOTS ( ( 4, 4 ),
 ( 0.6093138467282562809, 1.570796326794900111 ),
 .UNSPECIFIED. ) 
 CURVE ( )  GEOMETRIC_REPRESENTATION_ITEM ( )  RATIONAL_B_SPLINE_CURVE ( ( 1.000000000000000000, 0.9244349266169025192, 0.9244349266169025192, 1.000000000000000000 ) ) 
 REPRESENTATION_ITEM ( '' )  );
#26700=CIRCLE ( 'NONE', #10373, 7.461249999999999716 ) ;
#26707=CARTESIAN_POINT ( 'NONE',  ( -5.965356522962928842, 65.30181249999996851, 5.016499999999999737 ) ) ;
#26713=ORIENTED_EDGE ( 'NONE', *, *, #33225, .F. ) ;
#26728=CARTESIAN_POINT ( 'NONE',  ( 5.475330206976797953, 57.14999999999999858, -5.107412922131463695 ) ) ;
#26730=ORIENTED_EDGE ( 'NONE', *, *, #14115, .T. ) ;
#26741=AXIS2_PLACEMENT_3D ( 'NONE', #9819, #22785, #27012 ) ;
#26743=CARTESIAN_POINT ( 'NONE',  ( 4.792324638223571576, 56.51998046905274009, -4.972049999999996750 ) ) ;
#26744=ORIENTED_EDGE ( 'NONE', *, *, #3971, .F. ) ;
#26754=VECTOR ( 'NONE', #31257, 1000.000000000000000 ) ;
#26767=VERTEX_POINT ( 'NONE', #37825 ) ;
#26773=ORIENTED_EDGE ( 'NONE', *, *, #18254, .T. ) ;
#26777=DIRECTION ( 'NONE',  ( -0.9891443546370349837, 0.000000000000000000, 0.1469470846586743984 ) ) ;
#26782=CARTESIAN_POINT ( 'NONE',  ( 5.706393392168676471, 56.51499999999914792, 5.041882957346167871 ) ) ;
#26802=FACE_OUTER_BOUND ( 'NONE', #14545, .T. ) ;
#26804=DIRECTION ( 'NONE',  ( 1.000000000000000000, 0.000000000000000000, 0.000000000000000000 ) ) ;
#26821=CARTESIAN_POINT ( 'NONE',  ( -5.309060684617390516E-14, 83.56599999999998829, 0.000000000000000000 ) ) ;
#26830=CARTESIAN_POINT ( 'NONE',  ( 5.305748947172213015, 65.30181249999998272, -5.247078976224250013 ) ) ;
#26849=ORIENTED_EDGE ( 'NONE', *, *, #19865, .F. ) ;
#26857=DIRECTION ( 'NONE',  ( -1.000000000000000000, 9.627370216492862708E-17, 0.000000000000000000 ) ) ;
#26864=CARTESIAN_POINT ( 'NONE',  ( -5.230039278750650666, 78.94094791484918971, 5.321858878494039047 ) ) ;
#26865=CARTESIAN_POINT ( 'NONE',  ( -10.45722248778828423, 56.52709681235293715, -5.016499999999999737 ) ) ;
#26876=VERTEX_POINT ( 'NONE', #41034 ) ;
#26882=CARTESIAN_POINT ( 'NONE',  ( -23.49500000000000455, 71.11999999999999034, 1.904999999999985372 ) ) ;
#26894=CARTESIAN_POINT ( 'NONE',  ( 11.37822013471344995, 56.06794068206381354, -5.016500000000108983 ) ) ;
#26908=LINE ( 'NONE', #7536, #23957 ) ;
#26913=CARTESIAN_POINT ( 'NONE',  ( -17.14499999999999957, 71.11999999999999034, 5.016499999999999737 ) ) ;
#26920=EDGE_CURVE ( 'NONE', #17114, #30952, #25041, .T. ) ;
#26921=( BOUNDED_CURVE ( )  B_SPLINE_CURVE ( 3, ( #37317, #8134, #21107, #3915 ),
 .UNSPECIFIED., .F., .T. ) 
 B_SPLINE_CURVE_WITH_KNOTS ( ( 4, 4 ),
 ( 1.303225233037621953E-32, 1.570796326794896558 ),
 .UNSPECIFIED. ) 
 CURVE ( )  GEOMETRIC_REPRESENTATION_ITEM ( )  RATIONAL_B_SPLINE_CURVE ( ( 1.000000000000000000, 0.8047378541243649375, 0.8047378541243649375, 1.000000000000000000 ) ) 
 REPRESENTATION_ITEM ( '' )  );
#26922=EDGE_LOOP ( 'NONE', ( #37369, #39935, #14085, #25146, #37931, #37487, #25896, #5501 ) ) ;
#26936=AXIS2_PLACEMENT_3D ( 'NONE', #38090, #34065, #37248 ) ;
#26947=EDGE_CURVE ( 'NONE', #28739, #22885, #4854, .T. ) ;
#26969=DIRECTION ( 'NONE',  ( -0.1728608224830406603, -1.098208118798718614E-16, 0.9849462604886047856 ) ) ;
#26982=EDGE_CURVE ( 'NONE', #5344, #38115, #35698, .T. ) ;
#26987=FACE_OUTER_BOUND ( 'NONE', #15532, .T. ) ;
#26988=VERTEX_POINT ( 'NONE', #26094 ) ;
#27002=DIRECTION ( 'NONE',  ( -1.000000000000000000, 9.627370216492862708E-17, 0.000000000000000000 ) ) ;
#27003=VERTEX_POINT ( 'NONE', #6937 ) ;
#27006=CARTESIAN_POINT ( 'NONE',  ( -14.39766717389552220, 60.02151067229126369, 1.905000000000008686 ) ) ;
#27007=CIRCLE ( 'NONE', #3888, 6.349999999999999645 ) ;
#27012=DIRECTION ( 'NONE',  ( -1.000000000000000000, 0.000000000000000000, 0.000000000000000000 ) ) ;
#27015=VECTOR ( 'NONE', #4407, 1000.000000000000227 ) ;
#27039=CARTESIAN_POINT ( 'NONE',  ( 5.871452009091314039, 53.58606249999999704, -5.016499999999999737 ) ) ;
#27060=ORIENTED_EDGE ( 'NONE', *, *, #644, .T. ) ;
#27061=DIRECTION ( 'NONE',  ( -1.000000000000000000, 0.000000000000000000, 0.000000000000000000 ) ) ;
#27068=CARTESIAN_POINT ( 'NONE',  ( 1.589478822742971683E-15, 16.51000000000000156, 0.000000000000000000 ) ) ;
#27099=MECHANICAL_DESIGN_GEOMETRIC_PRESENTATION_REPRESENTATION('',(#6014),#30463);
#27121=CARTESIAN_POINT ( 'NONE',  ( -5.224225368397744873, 56.51499999999979451, 5.327462281792842091 ) ) ;
#27131=VERTEX_POINT ( 'NONE', #21778 ) ;
#27169=EDGE_CURVE ( 'NONE', #17039, #37617, #41579, .T. ) ;
#27173=CARTESIAN_POINT ( 'NONE',  ( -13.85159022459153988, 12.96416000000000146, 5.016499999999999737 ) ) ;
#27176=EDGE_LOOP ( 'NONE', ( #2044, #34838 ) ) ;
#27180=ORIENTED_EDGE ( 'NONE', *, *, #36377, .T. ) ;
#27187=VERTEX_POINT ( 'NONE', #16446 ) ;
#27195=VECTOR ( 'NONE', #14188, 1000.000000000000227 ) ;
#27245=CARTESIAN_POINT ( 'NONE',  ( 5.305748947172213015, 53.58606249999999704, -5.247078976224250013 ) ) ;
#27259=ORIENTED_EDGE ( 'NONE', *, *, #4058, .T. ) ;
#27269=CARTESIAN_POINT ( 'NONE',  ( 13.46199999999999797, 12.17394877578616708, 0.000000000000000000 ) ) ;
#27280=ORIENTED_EDGE ( 'NONE', *, *, #25909, .T. ) ;
#27285=CARTESIAN_POINT ( 'NONE',  ( -6.350000000000054712, 86.35999999999998522, 7.776507174585692163E-16 ) ) ;
#27298=CIRCLE ( 'NONE', #37508, 6.349999999999999645 ) ;
#27304=B_SPLINE_SURFACE_WITH_KNOTS ( 'NONE', 3, 1, ( 
 ( #22638, #36098 ),
 ( #3940, #740 ),
 ( #36511, #32682 ),
 ( #23274, #29266 ) ),
 .UNSPECIFIED., .F., .F., .F.,
 ( 4, 4 ),
 ( 2, 2 ),
 ( 0.000000000000000000, 0.6118630412642114269 ),
 ( 0.000000000000000000, 1.000000000000000000 ),
 .UNSPECIFIED. ) ;
#27315=CIRCLE ( 'NONE', #13726, 2.540000000000000480 ) ;
#27316=DIRECTION ( 'NONE',  ( -9.627370216492862708E-17, -1.000000000000000000, 0.000000000000000000 ) ) ;
#27323=AXIS2_PLACEMENT_3D ( 'NONE', #34719, #21280, #41330 ) ;
#27335=CARTESIAN_POINT ( 'NONE',  ( -4.781529118576368198, 56.51499999999999346, 4.872211946655436776 ) ) ;
#27362=EDGE_CURVE ( 'NONE', #2187, #4024, #25893, .T. ) ;
#27364=DIRECTION ( 'NONE',  ( 1.000000000000000000, 0.000000000000000000, -1.224646799147351728E-16 ) ) ;
#27365=ORIENTED_EDGE ( 'NONE', *, *, #13555, .F. ) ;
#27393=CARTESIAN_POINT ( 'NONE',  ( -6.073982626572030696, 78.87340550758391089, -4.346604155593818852 ) ) ;
#27396=ORIENTED_EDGE ( 'NONE', *, *, #14466, .T. ) ;
#27403=ORIENTED_EDGE ( 'NONE', *, *, #3466, .F. ) ;
#27412=ORIENTED_EDGE ( 'NONE', *, *, #39678, .F. ) ;
#27426=LINE ( 'NONE', #11231, #32176 ) ;
#27451=CARTESIAN_POINT ( 'NONE',  ( 10.19284229789036900, 16.51000000000000156, 4.908176479697702099 ) ) ;
#27456=CARTESIAN_POINT ( 'NONE',  ( 5.871452009091314039, 65.30181249999998272, -5.016499999999999737 ) ) ;
#27463=EDGE_CURVE ( 'NONE', #27491, #1397, #13478, .T. ) ;
#27465=ORIENTED_EDGE ( 'NONE', *, *, #39123, .F. ) ;
#27471=AXIS2_PLACEMENT_3D ( 'NONE', #23417, #20435, #16404 ) ;
#27491=VERTEX_POINT ( 'NONE', #506 ) ;
#27496=VECTOR ( 'NONE', #9756, 1000.000000000000000 ) ;
#27498=CYLINDRICAL_SURFACE ( 'NONE', #33841, 2.540000000000000480 ) ;
#27515=EDGE_LOOP ( 'NONE', ( #29058, #2852, #17557, #8902, #16605, #23021, #772 ) ) ;
#27525=VERTEX_POINT ( 'NONE', #23244 ) ;
#27530=CARTESIAN_POINT ( 'NONE',  ( 10.45888906141533603, 56.51500000000000057, -4.393716635382131308 ) ) ;
#27538=CARTESIAN_POINT ( 'NONE',  ( -12.21488373879589062, 55.24499999999999034, 5.016499999999999737 ) ) ;
#27547=CARTESIAN_POINT ( 'NONE',  ( -17.14499999999999957, 71.11999999999999034, 5.016499999999999737 ) ) ;
#27549=CARTESIAN_POINT ( 'NONE',  ( 5.137966006445083167, 56.84472104120887082, -5.330653870689105567 ) ) ;
#27563=CARTESIAN_POINT ( 'NONE',  ( 6.059261036834406866, 56.98375738874754859, 5.016500000000000625 ) ) ;
#27592=EDGE_LOOP ( 'NONE', ( #4420, #14411, #39200, #10052, #248, #23789, #20799, #24644 ) ) ;
#27597=CARTESIAN_POINT ( 'NONE',  ( 5.632494751982964232, 78.90911215162449821, -5.063853515469283195 ) ) ;
#27606=CARTESIAN_POINT ( 'NONE',  ( -7.461250000000054783, 85.80437499999999318, 9.137395930138188390E-16 ) ) ;
#27607=EDGE_LOOP ( 'NONE', ( #11401, #20586, #36412, #8259, #39507, #7419, #1386, #42031, #41959 ) ) ;
#27628=ADVANCED_FACE ( 'NONE', ( #4331 ), #39470, .F. ) ;
#27632=CARTESIAN_POINT ( 'NONE',  ( -12.21488373879589240, 12.96416000000000146, -4.381499999999999950 ) ) ;
#27644=DIRECTION ( 'NONE',  ( 1.224646799147353207E-16, -1.179012811983454535E-32, 1.000000000000000000 ) ) ;
#27646=AXIS2_PLACEMENT_3D ( 'NONE', #31059, #14650, #27654 ) ;
#27653=AXIS2_PLACEMENT_3D ( 'NONE', #38495, #35299, #6127 ) ;
#27654=DIRECTION ( 'NONE',  ( -1.000000000000000000, 0.000000000000000000, 0.000000000000000000 ) ) ;
#27665=ORIENTED_EDGE ( 'NONE', *, *, #23477, .T. ) ;
#27679=CARTESIAN_POINT ( 'NONE',  ( -5.305748947172282293, 57.14999999999999147, 5.247078976224250013 ) ) ;
#27688=EDGE_CURVE ( 'NONE', #18509, #31875, #27928, .T. ) ;
#27690=CARTESIAN_POINT ( 'NONE',  ( 10.28897677580357950, 56.51500000000000057, 5.016500000000000625 ) ) ;
#27714=ORIENTED_EDGE ( 'NONE', *, *, #23309, .F. ) ;
#27716=AXIS2_PLACEMENT_3D ( 'NONE', #37709, #21288, #1735 ) ;
#27723=DIRECTION ( 'NONE',  ( 0.1715592850456333085, 0.1224830539174543292, 0.9775302108976914317 ) ) ;
#27726=EDGE_CURVE ( 'NONE', #700, #18659, #17095, .T. ) ;
#27743=DIRECTION ( 'NONE',  ( 1.000000000000000000, 0.000000000000000000, 0.000000000000000000 ) ) ;
#27749=CARTESIAN_POINT ( 'NONE',  ( -14.73199999999999754, 61.59499999999999886, 5.016499999999999737 ) ) ;
#27755=EDGE_LOOP ( 'NONE', ( #1511, #32509, #9026, #31320, #2547, #29834, #12238 ) ) ;
#27765=VERTEX_POINT ( 'NONE', #20897 ) ;
#27767=CARTESIAN_POINT ( 'NONE',  ( 5.941785709847694719, 56.51500000000406487, 5.016499812911857425 ) ) ;
#27782=EDGE_CURVE ( 'NONE', #11710, #117, #34782, .T. ) ;
#27793=CARTESIAN_POINT ( 'NONE',  ( -12.21488373879589240, 17.14500000000000313, 5.016499999999999737 ) ) ;
#27815=ORIENTED_EDGE ( 'NONE', *, *, #1205, .F. ) ;
#27841=ADVANCED_FACE ( 'NONE', ( #37110 ), #17701, .F. ) ;
#27853=LINE ( 'NONE', #15272, #25117 ) ;
#27857=DIRECTION ( 'NONE',  ( -9.627370216492862708E-17, -1.000000000000000000, 0.000000000000000000 ) ) ;
#27879=ORIENTED_EDGE ( 'NONE', *, *, #40635, .F. ) ;
#27888=CARTESIAN_POINT ( 'NONE',  ( 6.059261036834405978, 56.51500000000000057, 4.381499999999999950 ) ) ;
#27892=CARTESIAN_POINT ( 'NONE',  ( -5.224239059777524119, 56.51499999999391122, -5.327449085208022517 ) ) ;
#27904=CARTESIAN_POINT ( 'NONE',  ( -11.58677707360137354, 55.24499999999998323, -4.474811398758258285 ) ) ;
#27913=EDGE_CURVE ( 'NONE', #4497, #24583, #27298, .T. ) ;
#27922=EDGE_CURVE ( 'NONE', #24940, #18746, #5167, .T. ) ;
#27928=LINE ( 'NONE', #5375, #11655 ) ;
#27939=VECTOR ( 'NONE', #10865, 1000.000000000000000 ) ;
#27951=DIRECTION ( 'NONE',  ( 0.000000000000000000, 0.000000000000000000, 1.000000000000000000 ) ) ;
#27952=DIRECTION ( 'NONE',  ( -9.627370216492862708E-17, -1.000000000000000000, 0.000000000000000000 ) ) ;
#27961=EDGE_CURVE ( 'NONE', #31875, #27131, #12998, .T. ) ;
#27996=LINE ( 'NONE', #25013, #39186 ) ;
#27998=VERTEX_POINT ( 'NONE', #9389 ) ;
#28013=CARTESIAN_POINT ( 'NONE',  ( 17.14499999999999957, 71.11999999999999034, -1.904999999999999583 ) ) ;
#28017=CARTESIAN_POINT ( 'NONE',  ( 16.60960244842765832, -1.599067919197793490E-15, 2.034089647357696937E-15 ) ) ;
#28021=CARTESIAN_POINT ( 'NONE',  ( 5.177913976931207252, 64.41499993257285439, -5.372100000000002318 ) ) ;
#28038=( BOUNDED_CURVE ( )  B_SPLINE_CURVE ( 3, ( #36027, #22997, #20649, #7268 ),
 .UNSPECIFIED., .F., .F. ) 
 B_SPLINE_CURVE_WITH_KNOTS ( ( 4, 4 ),
 ( 4.712388980384690562, 6.283185307179586232 ),
 .UNSPECIFIED. ) 
 CURVE ( )  GEOMETRIC_REPRESENTATION_ITEM ( )  RATIONAL_B_SPLINE_CURVE ( ( 1.000000000000000000, 0.8047378541243652705, 0.8047378541243652705, 1.000000000000000000 ) ) 
 REPRESENTATION_ITEM ( '' )  );
#28039=CARTESIAN_POINT ( 'NONE',  ( 4.880630303840320039, 56.51998046905275430, 4.886936331184463356 ) ) ;
#28050=CARTESIAN_POINT ( 'NONE',  ( 5.941750550382240093, 57.15000000000122071, -5.016499999999999737 ) ) ;
#28062=B_SPLINE_CURVE_WITH_KNOTS ( 'NONE', 3,
 ( #2209, #24339, #27549, #18782, #34785, #1787 ),
 .UNSPECIFIED., .F., .F.,
 ( 4, 2, 4 ),
 ( 0.000000000000000000, 0.4601069123252314874, 0.9202138246504629748 ),
 .UNSPECIFIED. ) ;
#28087=ORIENTED_EDGE ( 'NONE', *, *, #12698, .T. ) ;
#28096=DIRECTION ( 'NONE',  ( 0.9849462604886048966, -0.000000000000000000, 0.1728608224830406881 ) ) ;
#28104=CIRCLE ( 'NONE', #21316, 6.985000000000000320 ) ;
#28116=DIRECTION ( 'NONE',  ( -9.627370216492862708E-17, -1.000000000000000000, 0.000000000000000000 ) ) ;
#28133=ADVANCED_FACE ( 'NONE', ( #6993 ), #19962, .T. ) ;
#28136=LINE ( 'NONE', #15559, #2470 ) ;
#28153=CIRCLE ( 'NONE', #40428, 12.69999999999999751 ) ;
#28163=EDGE_CURVE ( 'NONE', #28739, #26298, #401, .T. ) ;
#28174=CARTESIAN_POINT ( 'NONE',  ( 10.86251533436112737, 78.45482716897194564, -1.904999999999999583 ) ) ;
#28186=ADVANCED_FACE ( 'NONE', ( #21943 ), #24572, .T. ) ;
#28218=CARTESIAN_POINT ( 'NONE',  ( -5.871452009091403745, 77.01756249999996840, -5.016499999999999737 ) ) ;
#28221=ORIENTED_EDGE ( 'NONE', *, *, #27782, .T. ) ;
#28230=DIRECTION ( 'NONE',  ( -1.000000000000000000, 0.000000000000000000, 0.000000000000000000 ) ) ;
#28233=CYLINDRICAL_SURFACE ( 'NONE', #14868, 2.540000000000000480 ) ;
#28264=AXIS2_PLACEMENT_3D ( 'NONE', #29335, #6140, #41711 ) ;
#28266=CARTESIAN_POINT ( 'NONE',  ( 5.256643466096790895, 56.51500000000020663, -5.296410793414215945 ) ) ;
#28268=DIRECTION ( 'NONE',  ( -6.353134868986658533E-16, 1.000000000000000000, 0.000000000000000000 ) ) ;
#28281=ORIENTED_EDGE ( 'NONE', *, *, #18506, .F. ) ;
#28284=DIRECTION ( 'NONE',  ( 0.000000000000000000, 0.000000000000000000, -1.000000000000000000 ) ) ;
#28286=CARTESIAN_POINT ( 'NONE',  ( -3.628388194583719468E-14, 57.78499999999999659, 1.904999999999999805 ) ) ;
#28289=CARTESIAN_POINT ( 'NONE',  ( 14.73199999999999577, 61.59499999999999886, 1.904999999999990479 ) ) ;
#28311=CARTESIAN_POINT ( 'NONE',  ( 13.85159022459153810, 60.48513866567135722, -5.016500000000000625 ) ) ;
#28312=CARTESIAN_POINT ( 'NONE',  ( 5.817775060672807363, 56.51500000000000057, 4.384522920466269014 ) ) ;
#28320=CARTESIAN_POINT ( 'NONE',  ( -10.86251533436120553, 78.45482716897194564, 1.904999999999999583 ) ) ;
#28334=CARTESIAN_POINT ( 'NONE',  ( -5.475330206976868119, 57.14999999999997016, -5.107412922131463695 ) ) ;
#28360=CARTESIAN_POINT ( 'NONE',  ( 10.28897677580358305, 57.15000000000000568, -4.381499999999999950 ) ) ;
#28365=ORIENTED_EDGE ( 'NONE', *, *, #16264, .T. ) ;
#28392=EDGE_LOOP ( 'NONE', ( #3521, #20324, #39097, #16073, #10475, #15467 ) ) ;
#28393=LINE ( 'NONE', #25194, #23633 ) ;
#28420=DIRECTION ( 'NONE',  ( -0.000000000000000000, -0.000000000000000000, -1.000000000000000000 ) ) ;
#28431=CARTESIAN_POINT ( 'NONE',  ( 12.69999999999999929, 17.14499999999999957, 1.555301434917138235E-15 ) ) ;
#28433=EDGE_CURVE ( 'NONE', #19034, #5073, #143, .T. ) ;
#28435=ORIENTED_EDGE ( 'NONE', *, *, #18057, .T. ) ;
#28439=VERTEX_POINT ( 'NONE', #11239 ) ;
#28452=FACE_OUTER_BOUND ( 'NONE', #28392, .T. ) ;
#28467=DIRECTION ( 'NONE',  ( 0.000000000000000000, 1.000000000000000000, 0.000000000000000000 ) ) ;
#28475=CYLINDRICAL_SURFACE ( 'NONE', #31373, 6.350000000000004974 ) ;
#28482=CARTESIAN_POINT ( 'NONE',  ( 5.423544988499409136, 78.92590603608628896, 5.135347845727595839 ) ) ;
#28499=EDGE_CURVE ( 'NONE', #11997, #1559, #23272, .T. ) ;
#28509=EDGE_LOOP ( 'NONE', ( #17239, #35438, #33535, #15852 ) ) ;
#28520=EDGE_LOOP ( 'NONE', ( #9759, #8138, #18365, #25543 ) ) ;
#28524=ADVANCED_FACE ( 'NONE', ( #16685 ), #19432, .T. ) ;
#28527=VECTOR ( 'NONE', #29762, 1000.000000000000000 ) ;
#28528=AXIS2_PLACEMENT_3D ( 'NONE', #4937, #24707, #8111 ) ;
#28530=CARTESIAN_POINT ( 'NONE',  ( -10.54112285291058981, 57.14999999999385949, 5.016499999999999737 ) ) ;
#28534=DIRECTION ( 'NONE',  ( -0.000000000000000000, -0.000000000000000000, -1.000000000000000000 ) ) ;
#28541=DIRECTION ( 'NONE',  ( 1.000000000000000000, 6.353134868986659519E-16, 0.000000000000000000 ) ) ;
#28545=CARTESIAN_POINT ( 'NONE',  ( 16.87828382557106721, 17.14499999999999957, -5.016499999999999737 ) ) ;
#28548=CARTESIAN_POINT ( 'NONE',  ( -4.792324638262678960, 56.51998046905272588, 4.972049999962470324 ) ) ;
#28578=CARTESIAN_POINT ( 'NONE',  ( 8.936628967501334841, 56.51500000000000057, 4.721553682181185430 ) ) ;
#28599=ORIENTED_EDGE ( 'NONE', *, *, #8734, .F. ) ;
#28605=B_SPLINE_CURVE_WITH_KNOTS ( 'NONE', 3,
 ( #22815, #26670, #35852, #18713, #3391, #16141, #2975, #2772, #15938, #3176, #18926, #12344, #34935, #32556, #2567, #25739 ),
 .UNSPECIFIED., .F., .F.,
 ( 4, 2, 2, 2, 2, 2, 2, 4 ),
 ( 0.000000000000000000, 0.2499999999999866773, 0.3749999999999802380, 0.4374999999999798495, 0.4687499999999812372, 0.4999999999999826805, 0.7499999999999913403, 1.000000000000000000 ),
 .UNSPECIFIED. ) ;
#28623=LINE ( 'NONE', #23047, #2296 ) ;
#28639=CARTESIAN_POINT ( 'NONE',  ( -5.664977208693910526, 88.73331249999999670, -5.033228321271210781 ) ) ;
#28642=ORIENTED_EDGE ( 'NONE', *, *, #15764, .F. ) ;
#28651=CARTESIAN_POINT ( 'NONE',  ( 10.39017547737320157, 56.51500000000000767, 4.336808689942017736E-15 ) ) ;
#28654=LINE ( 'NONE', #3744, #29841 ) ;
#28659=ORIENTED_EDGE ( 'NONE', *, *, #40635, .T. ) ;
#28674=DIRECTION ( 'NONE',  ( -0.1469470846586743706, 0.000000000000000000, 0.9891443546370348727 ) ) ;
#28678=CARTESIAN_POINT ( 'NONE',  ( -5.137966006445155109, 56.84472104120887792, 5.330653870689118001 ) ) ;
#28685=CARTESIAN_POINT ( 'NONE',  ( 5.706177858045066387, 56.51499999999918344, -5.041924731713509189 ) ) ;
#28689=ADVANCED_FACE ( 'NONE', ( #25854 ), #27304, .T. ) ;
#28695=CARTESIAN_POINT ( 'NONE',  ( -17.14499999999999957, 71.11999999999999034, -1.904999999999999583 ) ) ;
#28697=CARTESIAN_POINT ( 'NONE',  ( 6.059261036834405978, 56.51500000000000057, -4.547742611252458822 ) ) ;
#28704=CARTESIAN_POINT ( 'NONE',  ( -15.50061618130080987, 62.14374591690594940, 1.904999999999990035 ) ) ;
#28709=CARTESIAN_POINT ( 'NONE',  ( 5.638212235253492466, 56.51499999999996504, 5.060089761408623765 ) ) ;
#28725=CARTESIAN_POINT ( 'NONE',  ( 5.106395947886047004, 78.95054594174945350, 1.904999999999988258 ) ) ;
#28726=DIRECTION ( 'NONE',  ( 0.1728608224830406603, 0.000000000000000000, -0.9849462604886047856 ) ) ;
#28733=CARTESIAN_POINT ( 'NONE',  ( -11.66725022231030628, 55.24499999999999744, 5.016500000000000625 ) ) ;
#28737=CARTESIAN_POINT ( 'NONE',  ( -17.14499999999999957, 71.11999999999999034, 1.904999999999989146 ) ) ;
#28739=VERTEX_POINT ( 'NONE', #32469 ) ;
#28740=EDGE_LOOP ( 'NONE', ( #2378, #12719, #27665, #14126, #2448, #12713 ) ) ;
#28746=CARTESIAN_POINT ( 'NONE',  ( -5.451267667241070720E-14, 85.80437499999999318, 0.000000000000000000 ) ) ;
#28750=FACE_OUTER_BOUND ( 'NONE', #13421, .T. ) ;
#28751=CARTESIAN_POINT ( 'NONE',  ( -5.965356522962928842, 57.14999999999997016, -5.016499999999999737 ) ) ;
#28759=ORIENTED_EDGE ( 'NONE', *, *, #4350, .F. ) ;
#28767=VECTOR ( 'NONE', #1874, 1000.000000000000000 ) ;
#28768=ORIENTED_EDGE ( 'NONE', *, *, #32686, .F. ) ;
#28772=SHAPE_DEFINITION_REPRESENTATION ( #6879, #11484 ) ;
#28782=ORIENTED_EDGE ( 'NONE', *, *, #8720, .T. ) ;
#28786=AXIS2_PLACEMENT_3D ( 'NONE', #29863, #36054, #39244 ) ;
#28794=CIRCLE ( 'NONE', #22654, 0.6350000000000001199 ) ;
#28795=CARTESIAN_POINT ( 'NONE',  ( -5.177913976931285411, 57.14999999999999858, -5.372100000000001430 ) ) ;
#28805=CARTESIAN_POINT ( 'NONE',  ( -11.58677707360137532, 55.24499999999999034, -4.474811398758259173 ) ) ;
#28811=CARTESIAN_POINT ( 'NONE',  ( 5.664977208693820820, 65.30181249999998272, 5.033228321271210781 ) ) ;
#28831=ORIENTED_EDGE ( 'NONE', *, *, #9209, .T. ) ;
#28851=CARTESIAN_POINT ( 'NONE',  ( -6.059261036834474368, 65.30181249999998272, -5.016499999999999737 ) ) ;
#28890=CARTESIAN_POINT ( 'NONE',  ( 14.39766717389552220, 12.96416000000000146, 1.904999999999990923 ) ) ;
#28909=CARTESIAN_POINT ( 'NONE',  ( -14.39766717389552220, 60.02151067229126369, 1.905000000000008686 ) ) ;
#28927=FACE_OUTER_BOUND ( 'NONE', #2905, .T. ) ;
#28957=LINE ( 'NONE', #12772, #19461 ) ;
#28982=DIRECTION ( 'NONE',  ( -0.000000000000000000, -0.000000000000000000, -1.000000000000000000 ) ) ;
#28988=CARTESIAN_POINT ( 'NONE',  ( 10.92199999999999704, 55.24500000000000455, 0.000000000000000000 ) ) ;
#29004=DIRECTION ( 'NONE',  ( 0.000000000000000000, 1.000000000000000000, 0.000000000000000000 ) ) ;
#29005=CARTESIAN_POINT ( 'NONE',  ( 1.589478822742971486E-15, 16.51000000000000156, 0.000000000000000000 ) ) ;
#29009=ORIENTED_EDGE ( 'NONE', *, *, #31595, .F. ) ;
#29010=CARTESIAN_POINT ( 'NONE',  ( 6.059261036834406866, 53.58606249999999704, 5.016499999999999737 ) ) ;
#29025=DIRECTION ( 'NONE',  ( 0.000000000000000000, 0.000000000000000000, 1.000000000000000000 ) ) ;
#29043=CIRCLE ( 'NONE', #2560, 6.349999999999999645 ) ;
#29054=CARTESIAN_POINT ( 'NONE',  ( -5.241362157049125337, 53.58606249999999704, -5.310945289804168468 ) ) ;
#29058=ORIENTED_EDGE ( 'NONE', *, *, #19707, .T. ) ;
#29066=CARTESIAN_POINT ( 'NONE',  ( 5.348924234570989533, 56.51499999999999346, -4.492130288940734850 ) ) ;
#29070=CARTESIAN_POINT ( 'NONE',  ( -6.059261036834082681, 78.87450423423038615, 5.016499999999999737 ) ) ;
#29074=DIRECTION ( 'NONE',  ( 0.1469470846586743706, 9.335746474409589170E-17, 0.9891443546370348727 ) ) ;
#29085=VECTOR ( 'NONE', #24080, 1000.000000000000000 ) ;
#29088=EDGE_CURVE ( 'NONE', #700, #18747, #1157, .T. ) ;
#29095=CARTESIAN_POINT ( 'NONE',  ( 11.58677707360137532, 12.96416000000000146, 4.474811398758259173 ) ) ;
#29116=DIRECTION ( 'NONE',  ( 9.627370216492862708E-17, 1.000000000000000000, -0.000000000000000000 ) ) ;
#29122=CARTESIAN_POINT ( 'NONE',  ( -6.059261036834474368, 56.51499999999998636, -4.381499999999999950 ) ) ;
#29135=LINE ( 'NONE', #25733, #107 ) ;
#29148=CARTESIAN_POINT ( 'NONE',  ( -5.675123159882439872, 78.90545016724971106, -5.052246757648558351 ) ) ;
#29151=FACE_OUTER_BOUND ( 'NONE', #20152, .T. ) ;
#29156=AXIS2_PLACEMENT_3D ( 'NONE', #17265, #36032, #32833 ) ;
#29157=CARTESIAN_POINT ( 'NONE',  ( -5.309060684617390516E-14, 83.56599999999998829, 0.000000000000000000 ) ) ;
#29160=CARTESIAN_POINT ( 'NONE',  ( 16.87828382557106721, 17.14499999999999957, 5.016499999999999737 ) ) ;
#29178=EDGE_CURVE ( 'NONE', #21156, #25364, #35511, .T. ) ;
#29193=AXIS2_PLACEMENT_3D ( 'NONE', #28695, #18046, #11447 ) ;
#29197=ADVANCED_FACE ( 'NONE', ( #10719 ), #36720, .T. ) ;
#29198=FACE_OUTER_BOUND ( 'NONE', #36378, .T. ) ;
#29210=CARTESIAN_POINT ( 'NONE',  ( -3.590474171207809651E-14, 56.51499999999999346, 0.000000000000000000 ) ) ;
#29215=CARTESIAN_POINT ( 'NONE',  ( 5.177913976931196594, 78.94499979771845233, -5.372100000000001430 ) ) ;
#29222=CARTESIAN_POINT ( 'NONE',  ( 5.305748947172213015, 65.30181249999998272, 5.247078976224250013 ) ) ;
#29234=CARTESIAN_POINT ( 'NONE',  ( -14.60500000000000043, 71.11999999999999034, 5.016499999999999737 ) ) ;
#29240=EDGE_LOOP ( 'NONE', ( #39804, #40905, #25171, #27396 ) ) ;
#29243=ORIENTED_EDGE ( 'NONE', *, *, #38940, .T. ) ;
#29246=CARTESIAN_POINT ( 'NONE',  ( -13.85159022459153988, 59.63164443796365077, 5.016499999999999737 ) ) ;
#29248=CARTESIAN_POINT ( 'NONE',  ( 9.094996104468805243, 78.64197151092925253, -5.392902600000141433 ) ) ;
#29261=CARTESIAN_POINT ( 'NONE',  ( 11.66725022231030984, 17.14500000000046498, -5.016499999999999737 ) ) ;
#29265=CARTESIAN_POINT ( 'NONE',  ( -5.871452009091403745, 77.01756250000002524, 5.016499999999999737 ) ) ;
#29266=CARTESIAN_POINT ( 'NONE',  ( -5.106395947886143816, 78.95054594174945350, -5.392902600000144986 ) ) ;
#29288=CARTESIAN_POINT ( 'NONE',  ( -14.73199999999999399, 12.70000000000000462, 1.804149664503880250E-15 ) ) ;
#29309=ORIENTED_EDGE ( 'NONE', *, *, #26920, .F. ) ;
#29314=LINE ( 'NONE', #22475, #11662 ) ;
#29331=B_SPLINE_CURVE_WITH_KNOTS ( 'NONE', 3,
 ( #4321, #26453, #29861, #40308, #39456, #13672 ),
 .UNSPECIFIED., .F., .F.,
 ( 4, 2, 4 ),
 ( 0.0007477044786395083131, 0.001108740074962858389, 0.001469775671286208465 ),
 .UNSPECIFIED. ) ;
#29335=CARTESIAN_POINT ( 'NONE',  ( -17.14499999999999957, 71.11999999999999034, -1.904999999999999583 ) ) ;
#29349=AXIS2_PLACEMENT_3D ( 'NONE', #16210, #25602, #9416 ) ;
#29352=ORIENTED_EDGE ( 'NONE', *, *, #8411, .F. ) ;
#29359=CIRCLE ( 'NONE', #21769, 17.68910244842765778 ) ;
#29361=CARTESIAN_POINT ( 'NONE',  ( -5.322370864742718588, 56.51499999999976609, -5.239063871132868755 ) ) ;
#29368=CARTESIAN_POINT ( 'NONE',  ( -5.614623559985635559, 78.91041036408817888, -5.070733448224208573 ) ) ;
#29378=CARTESIAN_POINT ( 'NONE',  ( -6.059261036834476144, 56.98375738874752017, 5.016499999999999737 ) ) ;
#29382=CARTESIAN_POINT ( 'NONE',  ( -13.70915846191426191, 16.90875728684043011, -5.016499999999999737 ) ) ;
#29388=EDGE_LOOP ( 'NONE', ( #27412, #9682, #22024, #7095 ) ) ;
#29389=DIRECTION ( 'NONE',  ( -1.000000000000000000, -1.092739197465705287E-15, 0.000000000000000000 ) ) ;
#29397=ORIENTED_EDGE ( 'NONE', *, *, #13947, .F. ) ;
#29404=LINE ( 'NONE', #244, #2341 ) ;
#29409=DIRECTION ( 'NONE',  ( -1.000000000000000000, 0.000000000000000000, 0.000000000000000000 ) ) ;
#29410=CARTESIAN_POINT ( 'NONE',  ( 12.21488373879589240, 55.24500000000000455, 4.381499999999999950 ) ) ;
#29411=( BOUNDED_CURVE ( )  B_SPLINE_CURVE ( 3, ( #23294, #36332, #23720, #22870 ),
 .UNSPECIFIED., .F., .T. ) 
 B_SPLINE_CURVE_WITH_KNOTS ( ( 4, 4 ),
 ( 1.570796326794897890, 3.141592653589793116 ),
 .UNSPECIFIED. ) 
 CURVE ( )  GEOMETRIC_REPRESENTATION_ITEM ( )  RATIONAL_B_SPLINE_CURVE ( ( 1.000000000000000000, 0.8047378541243652705, 0.8047378541243652705, 1.000000000000000000 ) ) 
 REPRESENTATION_ITEM ( '' )  );
#29434=EDGE_CURVE ( 'NONE', #34925, #11069, #23257, .T. ) ;
#29439=CARTESIAN_POINT ( 'NONE',  ( 5.664977208693799504, 77.01756249999996840, 5.033228321271210781 ) ) ;
#29447=ORIENTED_EDGE ( 'NONE', *, *, #38940, .F. ) ;
#29457=EDGE_LOOP ( 'NONE', ( #37203, #1628 ) ) ;
#29466=PLANE ( 'NONE',  #36983 ) ;
#29474=CARTESIAN_POINT ( 'NONE',  ( -14.39766717389550266, 30.83083951148099189, 1.905000000000008686 ) ) ;
#29480=CARTESIAN_POINT ( 'NONE',  ( -5.177913976931283635, 53.58606250000000415, 5.372100000000000541 ) ) ;
#29487=CIRCLE ( 'NONE', #12493, 14.73199999999999577 ) ;
#29496=CARTESIAN_POINT ( 'NONE',  ( 10.92199999999999704, 55.24500000000000455, 0.000000000000000000 ) ) ;
#29523=LINE ( 'NONE', #28578, #22417 ) ;
#29525=VERTEX_POINT ( 'NONE', #11770 ) ;
#29528=CARTESIAN_POINT ( 'NONE',  ( -4.997525182441642677, 56.61525291752813160, 5.184946129310923801 ) ) ;
#29533=ADVANCED_FACE ( 'NONE', ( #6237 ), #2631, .F. ) ;
#29555=CARTESIAN_POINT ( 'NONE',  ( 9.925711944554072019, 78.55658865046544292, 5.016499999999999737 ) ) ;
#29560=CARTESIAN_POINT ( 'NONE',  ( 5.570730988718594290, 56.51499999999999346, 4.419918923950526768 ) ) ;
#29581=CARTESIAN_POINT ( 'NONE',  ( -5.936184715466119144, 56.51499999999997925, -4.381499802639526209 ) ) ;
#29601=DIRECTION ( 'NONE',  ( 1.776356839400250465E-15, 0.000000000000000000, 1.000000000000000000 ) ) ;
#29643=CARTESIAN_POINT ( 'NONE',  ( -10.28897677580358128, 56.51499999999998636, -5.016500000000000625 ) ) ;
#29652=ORIENTED_EDGE ( 'NONE', *, *, #32611, .T. ) ;
#29660=ORIENTED_EDGE ( 'NONE', *, *, #27961, .T. ) ;
#29664=DIRECTION ( 'NONE',  ( 1.000000000000000000, -5.463695987328526437E-16, -0.000000000000000000 ) ) ;
#29665=( BOUNDED_CURVE ( )  B_SPLINE_CURVE ( 3, ( #30203, #4244, #14008, #40023 ),
 .UNSPECIFIED., .F., .T. ) 
 B_SPLINE_CURVE_WITH_KNOTS ( ( 4, 4 ),
 ( 3.750906500318049286, 4.712388980384690562 ),
 .UNSPECIFIED. ) 
 CURVE ( )  GEOMETRIC_REPRESENTATION_ITEM ( )  RATIONAL_B_SPLINE_CURVE ( ( 1.000000000000000000, 0.9244349266169029633, 0.9244349266169029633, 1.000000000000000000 ) ) 
 REPRESENTATION_ITEM ( '' )  );
#29682=CARTESIAN_POINT ( 'NONE',  ( -10.28897677580358305, 56.51499999999998636, 5.016500000000000625 ) ) ;
#29689=CARTESIAN_POINT ( 'NONE',  ( 10.92199999999999704, 55.24500000000000455, 3.904382278571533962E-15 ) ) ;
#29696=ORIENTED_EDGE ( 'NONE', *, *, #23992, .T. ) ;
#29710=CARTESIAN_POINT ( 'NONE',  ( 5.664977208693820820, 57.14999999999999858, -5.033228321271210781 ) ) ;
#29725=ORIENTED_EDGE ( 'NONE', *, *, #39925, .T. ) ;
#29729=CARTESIAN_POINT ( 'NONE',  ( -12.21488373879589240, 55.24499999999999034, 4.381499999999999950 ) ) ;
#29731=ADVANCED_FACE ( 'NONE', ( #15590 ), #9219, .F. ) ;
#29734=CARTESIAN_POINT ( 'NONE',  ( -5.177913976931290740, 56.99702125087954130, -5.372099999999995212 ) ) ;
#29757=ORIENTED_EDGE ( 'NONE', *, *, #36023, .F. ) ;
#29762=DIRECTION ( 'NONE',  ( 1.000000000000000000, -9.627370216492862708E-17, 0.000000000000000000 ) ) ;
#29765=EDGE_CURVE ( 'NONE', #4305, #21064, #30755, .T. ) ;
#29780=ORIENTED_EDGE ( 'NONE', *, *, #38069, .T. ) ;
#29782=CARTESIAN_POINT ( 'NONE',  ( -9.094996104468895837, 78.64197151092922411, 5.392902600000138769 ) ) ;
#29783=CARTESIAN_POINT ( 'NONE',  ( 14.91798719394653894, 12.51401280605345789, 0.000000000000000000 ) ) ;
#29788=CARTESIAN_POINT ( 'NONE',  ( 11.41714695485569919, 57.15000000000000568, -5.016500000000000625 ) ) ;
#29795=CARTESIAN_POINT ( 'NONE',  ( -5.177913976931298734, 78.94499979771843812, -5.372100000000003206 ) ) ;
#29796=ADVANCED_FACE ( 'NONE', ( #6653 ), #19617, .F. ) ;
#29800=EDGE_CURVE ( 'NONE', #29525, #22768, #1531, .T. ) ;
#29812=EDGE_CURVE ( 'NONE', #34762, #14687, #25213, .T. ) ;
#29822=ORIENTED_EDGE ( 'NONE', *, *, #33529, .T. ) ;
#29834=ORIENTED_EDGE ( 'NONE', *, *, #35443, .T. ) ;
#29837=DIRECTION ( 'NONE',  ( -1.000000000000000000, 0.000000000000000000, 0.000000000000000000 ) ) ;
#29841=VECTOR ( 'NONE', #25668, 1000.000000000000000 ) ;
#29843=CARTESIAN_POINT ( 'NONE',  ( 11.97180806971946865, 56.20439414706014958, 5.016499999999999737 ) ) ;
#29850=CARTESIAN_POINT ( 'NONE',  ( -6.059261036834082681, 78.87450423423038615, 5.016499999999999737 ) ) ;
#29854=DIRECTION ( 'NONE',  ( -6.353134868986659519E-16, 1.000000000000000000, -0.000000000000000000 ) ) ;
#29861=CARTESIAN_POINT ( 'NONE',  ( -5.578816284158369498, 56.51500000000002188, 4.418322536902429043 ) ) ;
#29863=CARTESIAN_POINT ( 'NONE',  ( 17.14500000000001023, 57.15000000000000568, 4.381499999999999950 ) ) ;
#29870=VERTEX_POINT ( 'NONE', #16427 ) ;
#29875=CIRCLE ( 'NONE', #4715, 2.540000000000000480 ) ;
#29894=AXIS2_PLACEMENT_3D ( 'NONE', #32159, #6185, #35991 ) ;
#29906=VERTEX_POINT ( 'NONE', #32845 ) ;
#29922=VERTEX_POINT ( 'NONE', #29215 ) ;
#29934=ORIENTED_EDGE ( 'NONE', *, *, #9933, .T. ) ;
#29937=DIRECTION ( 'NONE',  ( -1.000000000000000000, 1.288607544181256449E-16, 0.000000000000000000 ) ) ;
#29965=DIRECTION ( 'NONE',  ( 0.1469470846586743706, 0.000000000000000000, 0.9891443546370348727 ) ) ;
#29981=CARTESIAN_POINT ( 'NONE',  ( 1.589478822742971683E-15, 16.51000000000000156, 0.000000000000000000 ) ) ;
#29992=CYLINDRICAL_SURFACE ( 'NONE', #32172, 7.461249999999999716 ) ;
#30001=PRODUCT ( 'Corkscrew Body', 'Corkscrew Body', '', ( #32814 ) ) ;
#30013=CARTESIAN_POINT ( 'NONE',  ( 15.50061618130081165, 62.14374591690594940, 1.904999999999990035 ) ) ;
#30019=CARTESIAN_POINT ( 'NONE',  ( 5.177913976931216133, 53.58606249999999704, -5.372100000000000541 ) ) ;
#30043=AXIS2_PLACEMENT_3D ( 'NONE', #38063, #31668, #8880 ) ;
#30050=EDGE_CURVE ( 'NONE', #17039, #22739, #41523, .T. ) ;
#30058=CARTESIAN_POINT ( 'NONE',  ( -5.565035070531761718, 78.91452218770618288, 5.089667964246479492 ) ) ;
#30069=EDGE_CURVE ( 'NONE', #3380, #5970, #14562, .T. ) ;
#30098=EDGE_CURVE ( 'NONE', #6334, #926, #19194, .T. ) ;
#30146=EDGE_LOOP ( 'NONE', ( #12554, #2359, #14711, #27403 ) ) ;
#30154=CIRCLE ( 'NONE', #13154, 14.73199999999999577 ) ;
#30160=CARTESIAN_POINT ( 'NONE',  ( 5.177913976931212581, 57.15000000000004832, -5.372100000000001430 ) ) ;
#30161=CIRCLE ( 'NONE', #13164, 6.350000000000004974 ) ;
#30187=ORIENTED_EDGE ( 'NONE', *, *, #30555, .T. ) ;
#30203=CARTESIAN_POINT ( 'NONE',  ( -14.39766717389552397, 60.02151067229126369, -1.904999999999999805 ) ) ;
#30204=AXIS2_PLACEMENT_3D ( 'NONE', #8946, #18510, #2146 ) ;
#30211=CARTESIAN_POINT ( 'NONE',  ( -3.630816577625875226E-14, 57.14999999999999147, 0.000000000000000000 ) ) ;
#30228=CARTESIAN_POINT ( 'NONE',  ( 5.241362157049035631, 77.01756249999996840, -5.310945289804168468 ) ) ;
#30251=DIRECTION ( 'NONE',  ( -1.000000000000000000, -1.004817652842027660E-15, -1.776356839400250465E-15 ) ) ;
#30280=EDGE_CURVE ( 'NONE', #3167, #11643, #38352, .T. ) ;
#30295=CARTESIAN_POINT ( 'NONE',  ( 11.66725022231030984, 55.24499999999999744, -5.016500000000003290 ) ) ;
#30314=CARTESIAN_POINT ( 'NONE',  ( 6.057513928997552810, 83.56599999999998829, 1.904999999999996030 ) ) ;
#30320=EDGE_CURVE ( 'NONE', #31705, #5725, #34952, .T. ) ;
#30360=CARTESIAN_POINT ( 'NONE',  ( 5.177913976931214357, 57.15000000000004832, 5.372099999999999653 ) ) ;
#30379=LINE ( 'NONE', #14394, #36052 ) ;
#30382=EDGE_CURVE ( 'NONE', #26767, #33803, #5775, .T. ) ;
#30425=B_SPLINE_CURVE_WITH_KNOTS ( 'NONE', 3,
 ( #9156, #11707, #24479, #12347, #8523, #34514 ),
 .UNSPECIFIED., .F., .F.,
 ( 4, 2, 4 ),
 ( 0.000000000000000000, 0.5000000000000000000, 1.000000000000000000 ),
 .UNSPECIFIED. ) ;
#30449=EDGE_LOOP ( 'NONE', ( #7185, #41313, #11109, #14301, #29780, #14726 ) ) ;
#30462=FACE_OUTER_BOUND ( 'NONE', #40684, .T. ) ;
#30463=( GEOMETRIC_REPRESENTATION_CONTEXT ( 3 ) GLOBAL_UNCERTAINTY_ASSIGNED_CONTEXT ( ( #20142 ) ) GLOBAL_UNIT_ASSIGNED_CONTEXT ( ( #38995, #35375, #9387 ) ) REPRESENTATION_CONTEXT ( 'NONE', 'WORKASPACE' ) );
#30465=CARTESIAN_POINT ( 'NONE',  ( -3.671158984043940170E-14, 57.78499999999999659, 0.000000000000000000 ) ) ;
#30478=CARTESIAN_POINT ( 'NONE',  ( -5.241362157049126225, 57.14999999999997016, -5.310945289804168468 ) ) ;
#30481=EDGE_CURVE ( 'NONE', #33118, #19034, #4965, .T. ) ;
#30490=EDGE_LOOP ( 'NONE', ( #11496, #11275, #34747, #16301 ) ) ;
#30496=CARTESIAN_POINT ( 'NONE',  ( 5.382937502775954980E-14, 83.56599999999998829, -1.904999999999999805 ) ) ;
#30506=CARTESIAN_POINT ( 'NONE',  ( 10.94257363143046291, 56.35470871607773802, -4.428493390991016021 ) ) ;
#30531=ORIENTED_EDGE ( 'NONE', *, *, #9457, .F. ) ;
#30539=CIRCLE ( 'NONE', #12179, 13.46199999999999619 ) ;
#30555=EDGE_CURVE ( 'NONE', #20294, #25746, #20437, .T. ) ;
#30564=CYLINDRICAL_SURFACE ( 'NONE', #16352, 2.540000000000000480 ) ;
#30594=AXIS2_PLACEMENT_3D ( 'NONE', #11174, #10964, #31772 ) ;
#30595=DIRECTION ( 'NONE',  ( 0.000000000000000000, 0.000000000000000000, 1.000000000000000000 ) ) ;
#30598=VECTOR ( 'NONE', #26139, 1000.000000000000000 ) ;
#30612=DIRECTION ( 'NONE',  ( 1.000000000000000000, 0.000000000000000000, -6.146657985744592735E-16 ) ) ;
#30617=DIRECTION ( 'NONE',  ( 9.627370216492862708E-17, 1.000000000000000000, -0.000000000000000000 ) ) ;
#30620=DIRECTION ( 'NONE',  ( 6.353134868986659519E-16, -1.000000000000000000, 0.000000000000000000 ) ) ;
#30628=EDGE_LOOP ( 'NONE', ( #14600, #2145, #17696, #15386, #35843 ) ) ;
#30646=CARTESIAN_POINT ( 'NONE',  ( 5.305748947172191698, 77.01756249999996840, -5.247078976224250013 ) ) ;
#30701=CARTESIAN_POINT ( 'NONE',  ( 16.42052266156670726, 59.67959903468464233, 5.072843609925764774 ) ) ;
#30704=AXIS2_PLACEMENT_3D ( 'NONE', #19335, #12746, #9548 ) ;
#30711=CIRCLE ( 'NONE', #19150, 14.73199999999999577 ) ;
#30712=CARTESIAN_POINT ( 'NONE',  ( 11.47253659098496925, 56.76836532675937974, -5.016500000000000625 ) ) ;
#30722=CARTESIAN_POINT ( 'NONE',  ( -10.79307885933852340, 57.10041794475175436, 5.016499999999999737 ) ) ;
#30739=EDGE_LOOP ( 'NONE', ( #39821, #14204, #8287, #23444 ) ) ;
#30748=ORIENTED_EDGE ( 'NONE', *, *, #6109, .F. ) ;
#30755=CIRCLE ( 'NONE', #34184, 12.69999999999999751 ) ;
#30763=VECTOR ( 'NONE', #28420, 1000.000000000000000 ) ;
#30764=CARTESIAN_POINT ( 'NONE',  ( 19.68500000000000227, 71.11999999999999034, 5.016499999999999737 ) ) ;
#30775=AXIS2_PLACEMENT_3D ( 'NONE', #16272, #16909, #13085 ) ;
#30788=CARTESIAN_POINT ( 'NONE',  ( 5.540303739757897361, 78.91648400349126291, -5.100389098699506185 ) ) ;
#30796=EDGE_LOOP ( 'NONE', ( #11599, #19575, #23679, #27465, #38431, #40274, #11876, #20238, #21762, #15508, #5634, #19856 ) ) ;
#30807=EDGE_CURVE ( 'NONE', #26988, #36287, #6186, .T. ) ;
#30820=DIRECTION ( 'NONE',  ( 1.000000000000000000, 6.353134868986659519E-16, 0.000000000000000000 ) ) ;
#30842=DIRECTION ( 'NONE',  ( 0.000000000000000000, 0.000000000000000000, -1.000000000000000000 ) ) ;
#30850=DIRECTION ( 'NONE',  ( -0.1469470846586743706, 0.000000000000000000, 0.9891443546370348727 ) ) ;
#30854=CARTESIAN_POINT ( 'NONE',  ( 5.475330206976777525, 88.73331249999999670, -5.107412922131463695 ) ) ;
#30877=APPLICATION_CONTEXT ( 'automotive_design' ) ;
#30878=CIRCLE ( 'NONE', #9808, 18.32410244842765934 ) ;
#30912=ORIENTED_EDGE ( 'NONE', *, *, #39433, .T. ) ;
#30913=ORIENTED_EDGE ( 'NONE', *, *, #7649, .T. ) ;
#30924=EDGE_LOOP ( 'NONE', ( #14811, #37981, #28087, #18700 ) ) ;
#30927=EDGE_LOOP ( 'NONE', ( #21037, #25455, #26730, #23, #33703, #27365, #16482, #38028, #7104, #38628, #12845 ) ) ;
#30929=DIRECTION ( 'NONE',  ( 0.000000000000000000, 1.000000000000000000, 0.000000000000000000 ) ) ;
#30941=CARTESIAN_POINT ( 'NONE',  ( -6.059261036834482361, 64.39150124418098642, -5.016499999999999737 ) ) ;
#30952=VERTEX_POINT ( 'NONE', #4155 ) ;
#31005=VERTEX_POINT ( 'NONE', #36521 ) ;
#31007=ORIENTED_EDGE ( 'NONE', *, *, #12028, .F. ) ;
#31022=AXIS2_PLACEMENT_3D ( 'NONE', #11502, #2150, #21702 ) ;
#31028=CARTESIAN_POINT ( 'NONE',  ( 10.92199999999999704, 55.24500000000000455, -3.904382278571533962E-15 ) ) ;
#31029=DIRECTION ( 'NONE',  ( -0.000000000000000000, -0.000000000000000000, -1.000000000000000000 ) ) ;
#31036=CARTESIAN_POINT ( 'NONE',  ( 5.511275327877898533, 57.15000000000044622, -5.111309965977538283 ) ) ;
#31038=CARTESIAN_POINT ( 'NONE',  ( 5.177913976931214357, 57.15000000000004832, 5.372099999999999653 ) ) ;
#31040=ADVANCED_FACE ( 'NONE', ( #32477, #23073 ), #6708, .T. ) ;
#31053=EDGE_LOOP ( 'NONE', ( #34545, #17710, #4440, #41358, #619 ) ) ;
#31056=DIRECTION ( 'NONE',  ( 0.000000000000000000, -1.000000000000000000, 0.000000000000000000 ) ) ;
#31059=CARTESIAN_POINT ( 'NONE',  ( -5.309060684617390516E-14, 83.56599999999998829, 0.000000000000000000 ) ) ;
#31075=EDGE_LOOP ( 'NONE', ( #36941, #1313, #22400, #29757 ) ) ;
#31076=CIRCLE ( 'NONE', #10671, 0.6350000000000001199 ) ;
#31078=ORIENTED_EDGE ( 'NONE', *, *, #11250, .F. ) ;
#31088=VECTOR ( 'NONE', #31193, 1000.000000000000000 ) ;
#31090=EDGE_CURVE ( 'NONE', #2471, #11710, #11777, .T. ) ;
#31096=ORIENTED_EDGE ( 'NONE', *, *, #21909, .F. ) ;
#31099=EDGE_CURVE ( 'NONE', #17114, #21064, #36942, .T. ) ;
#31103=CARTESIAN_POINT ( 'NONE',  ( -11.55299880265461887, 55.57741982016710125, -4.472382752598250910 ) ) ;
#31109=CARTESIAN_POINT ( 'NONE',  ( -19.68500000000000227, 71.11999999999999034, 5.016499999999999737 ) ) ;
#31121=ORIENTED_EDGE ( 'NONE', *, *, #30382, .T. ) ;
#31131=CARTESIAN_POINT ( 'NONE',  ( -3.671158984043940170E-14, 57.78499999999999659, 0.000000000000000000 ) ) ;
#31185=CARTESIAN_POINT ( 'NONE',  ( -3.628388194583719468E-14, 57.78499999999999659, 1.904999999999999805 ) ) ;
#31188=LINE ( 'NONE', #41218, #11294 ) ;
#31193=DIRECTION ( 'NONE',  ( 0.000000000000000000, 1.000000000000000000, 0.000000000000000000 ) ) ;
#31206=CARTESIAN_POINT ( 'NONE',  ( 7.213960532363567602, 83.56599999999998829, 1.904999999999995364 ) ) ;
#31227=AXIS2_PLACEMENT_3D ( 'NONE', #25024, #8847, #2474 ) ;
#31229=CIRCLE ( 'NONE', #25118, 7.461249999999999716 ) ;
#31230=CARTESIAN_POINT ( 'NONE',  ( 13.77279150232676130, 16.85108474679722690, -5.016499999999997961 ) ) ;
#31241=CARTESIAN_POINT ( 'NONE',  ( 5.638141748386683361, 56.51499999999961688, -5.060111600422207090 ) ) ;
#31249=LINE ( 'NONE', #8478, #4345 ) ;
#31252=CIRCLE ( 'NONE', #25814, 16.60960244842765832 ) ;
#31257=DIRECTION ( 'NONE',  ( 9.627370216492862708E-17, 1.000000000000000000, -0.000000000000000000 ) ) ;
#31282=B_SPLINE_CURVE_WITH_KNOTS ( 'NONE', 3,
 ( #31460, #31677, #3510, #16680, #6904, #12080, #18670, #2517, #28482, #23267 ),
 .UNSPECIFIED., .F., .F.,
 ( 4, 2, 2, 2, 4 ),
 ( 0.007397145391538724121, 0.008407694387831695856, 0.009418243384124665857, 0.01042879238041763759, 0.01143934137671060933 ),
 .UNSPECIFIED. ) ;
#31295=CARTESIAN_POINT ( 'NONE',  ( 10.28897677580357950, 56.51500000000000057, 4.381499999999999950 ) ) ;
#31306=CARTESIAN_POINT ( 'NONE',  ( -11.48503488083589730, 55.92196062030022574, -5.016499999999890491 ) ) ;
#31320=ORIENTED_EDGE ( 'NONE', *, *, #11735, .F. ) ;
#31327=ORIENTED_EDGE ( 'NONE', *, *, #5930, .T. ) ;
#31337=DIRECTION ( 'NONE',  ( -1.000000000000000000, 0.000000000000000000, 0.000000000000000000 ) ) ;
#31338=AXIS2_PLACEMENT_3D ( 'NONE', #2857, #29025, #41840 ) ;
#31369=ORIENTED_EDGE ( 'NONE', *, *, #15522, .F. ) ;
#31371=ORIENTED_EDGE ( 'NONE', *, *, #18005, .F. ) ;
#31373=AXIS2_PLACEMENT_3D ( 'NONE', #21844, #31029, #31451 ) ;
#31380=EDGE_CURVE ( 'NONE', #15239, #9633, #22185, .T. ) ;
#31385=DIRECTION ( 'NONE',  ( 0.1728608224830406603, 0.000000000000000000, -0.9849462604886047856 ) ) ;
#31395=AXIS2_PLACEMENT_3D ( 'NONE', #31471, #30842, #15064 ) ;
#31424=CARTESIAN_POINT ( 'NONE',  ( 5.285751105924014759, 78.93631598568867958, -5.267410652559297191 ) ) ;
#31428=FACE_OUTER_BOUND ( 'NONE', #29388, .T. ) ;
#31444=AXIS2_PLACEMENT_3D ( 'NONE', #10923, #23913, #36929 ) ;
#31451=DIRECTION ( 'NONE',  ( -1.000000000000000000, 0.000000000000000000, 0.000000000000000000 ) ) ;
#31458=CARTESIAN_POINT ( 'NONE',  ( 5.322311914403613287, 56.51499999999978030, -5.239113282919442227 ) ) ;
#31460=CARTESIAN_POINT ( 'NONE',  ( 7.213960532367366341, 78.77618639008778700, 1.904999999999999583 ) ) ;
#31465=EDGE_LOOP ( 'NONE', ( #17836, #8778, #5163, #41708, #1242 ) ) ;
#31471=CARTESIAN_POINT ( 'NONE',  ( 17.14499999999999957, 71.11999999999999034, -1.904999999999999583 ) ) ;
#31476=CARTESIAN_POINT ( 'NONE',  ( 7.127785904777375059, 78.78377652171666057, -2.231330898844071875 ) ) ;
#31501=DIRECTION ( 'NONE',  ( -1.000000000000000000, 0.000000000000000000, 0.000000000000000000 ) ) ;
#31507=CARTESIAN_POINT ( 'NONE',  ( -11.37822013471369864, 56.06794068206548332, 5.016500000000540638 ) ) ;
#31510=DIRECTION ( 'NONE',  ( -6.353134868986659519E-16, 1.000000000000000000, 0.000000000000000000 ) ) ;
#31520=CARTESIAN_POINT ( 'NONE',  ( -12.21488373878702127, 55.49440886859285627, -5.016499999999999737 ) ) ;
#31522=AXIS2_PLACEMENT_3D ( 'NONE', #29981, #20797, #27002 ) ;
#31525=CARTESIAN_POINT ( 'NONE',  ( 15.36699999999999733, 12.96302561210691628, 1.881914736249736896E-15 ) ) ;
#31529=DIRECTION ( 'NONE',  ( -0.000000000000000000, -0.000000000000000000, -1.000000000000000000 ) ) ;
#31545=CARTESIAN_POINT ( 'NONE',  ( 8.689997779576109740E-16, 9.026346327358515609, 0.000000000000000000 ) ) ;
#31550=DIRECTION ( 'NONE',  ( 9.627370216492862708E-17, 1.000000000000000000, -0.000000000000000000 ) ) ;
#31559=DIRECTION ( 'NONE',  ( -0.000000000000000000, -0.000000000000000000, -1.000000000000000000 ) ) ;
#31572=PRODUCT_DEFINITION ( 'UNKNOWN', '', #8708, #22694 ) ;
#31577=AXIS2_PLACEMENT_3D ( 'NONE', #22872, #25472, #6932 ) ;
#31583=CARTESIAN_POINT ( 'NONE',  ( 6.059261036834406866, 57.14999999999999858, 5.016499999999999737 ) ) ;
#31587=EDGE_LOOP ( 'NONE', ( #38682, #37703, #27879, #4531 ) ) ;
#31590=VERTEX_POINT ( 'NONE', #35847 ) ;
#31595=EDGE_CURVE ( 'NONE', #39783, #19939, #6867, .T. ) ;
#31620=ADVANCED_FACE ( 'NONE', ( #20254 ), #6448, .T. ) ;
#31621=DIRECTION ( 'NONE',  ( 0.000000000000000000, -0.000000000000000000, -1.000000000000000000 ) ) ;
#31634=VERTEX_POINT ( 'NONE', #39459 ) ;
#31639=CARTESIAN_POINT ( 'NONE',  ( 5.555120986090499535, 78.91530963298721701, -5.093895734005235099 ) ) ;
#31662=DIRECTION ( 'NONE',  ( -9.627370216492862708E-17, -1.000000000000000000, 0.000000000000000000 ) ) ;
#31668=DIRECTION ( 'NONE',  ( 9.627370216492862708E-17, 1.000000000000000000, -0.000000000000000000 ) ) ;
#31675=CARTESIAN_POINT ( 'NONE',  ( 5.449044798931634404, 57.15000000000252811, -5.145813327217715560 ) ) ;
#31677=CARTESIAN_POINT ( 'NONE',  ( 7.126949251439474331, 78.78385021288468693, 2.234499184491886670 ) ) ;
#31705=VERTEX_POINT ( 'NONE', #39885 ) ;
#31721=CARTESIAN_POINT ( 'NONE',  ( -4.825844303143389524, 56.51499999999997215, -4.829557277217701561 ) ) ;
#31722=CARTESIAN_POINT ( 'NONE',  ( -11.08653569745463052, 56.26057688450561045, 4.438844214435411217 ) ) ;
#31726=CARTESIAN_POINT ( 'NONE',  ( -15.15189561879767410, 77.97492127061565270, 1.904999999999999583 ) ) ;
#31739=CARTESIAN_POINT ( 'NONE',  ( -6.059261036834476144, 57.14999999999999858, -5.016499999999999737 ) ) ;
#31743=CARTESIAN_POINT ( 'NONE',  ( -4.880629475884273205, 56.51998046905272588, 4.886937129211982977 ) ) ;
#31770=ORIENTED_EDGE ( 'NONE', *, *, #27726, .F. ) ;
#31772=DIRECTION ( 'NONE',  ( -1.000000000000000000, -6.353134868986659519E-16, 0.000000000000000000 ) ) ;
#31782=CARTESIAN_POINT ( 'NONE',  ( -5.177913976931296069, 71.67999986514567468, -5.372099999999999653 ) ) ;
#31809=ORIENTED_EDGE ( 'NONE', *, *, #36608, .T. ) ;
#31827=EDGE_CURVE ( 'NONE', #27525, #22696, #37634, .T. ) ;
#31832=ORIENTED_EDGE ( 'NONE', *, *, #24317, .T. ) ;
#31837=CARTESIAN_POINT ( 'NONE',  ( -6.059261036834497460, 77.01756249999996840, -5.016499999999999737 ) ) ;
#31849=CARTESIAN_POINT ( 'NONE',  ( 6.059261036834406866, 57.14999999999999858, -5.016499999999999737 ) ) ;
#31850=CIRCLE ( 'NONE', #10075, 18.32410244842765934 ) ;
#31872=DIRECTION ( 'NONE',  ( -0.9891443546370349837, 0.000000000000000000, -0.1469470846586743984 ) ) ;
#31875=VERTEX_POINT ( 'NONE', #17 ) ;
#31881=CARTESIAN_POINT ( 'NONE',  ( -14.60500000000000043, 71.11999999999999034, 5.016499999999999737 ) ) ;
#31884=B_SPLINE_CURVE_WITH_KNOTS ( 'NONE', 3,
 ( #5457, #2049, #31424, #25030, #8853, #21817, #34843, #5677, #30788, #31639, #24184, #8015, #14592, #27597, #11406, #22442, #12470, #25465, #12675, #25664, #6294, #9891, #125, #38671 ),
 .UNSPECIFIED., .F., .F.,
 ( 4, 2, 2, 2, 1, 2, 2, 2, 2, 1, 2, 2, 4 ),
 ( 0.000000000000000000, 0.2499999999999528155, 0.3749999999999274469, 0.4374999999999140687, 0.4687499999999092948, 0.4843749999999090172, 0.4999999999999087397, 0.6249999999999164002, 0.6874999999999221734, 0.7187499999999252820, 0.7343749999999282796, 0.7499999999999311662, 1.000000000000000000 ),
 .UNSPECIFIED. ) ;
#31894=( BOUNDED_SURFACE ( )  B_SPLINE_SURFACE ( 3, 2, ( 
 ( #13152, #22295, #42143 ),
 ( #19323, #32327, #25515 ),
 ( #3156, #38935, #34904 ),
 ( #16336, #9746, #38307 ),
 ( #26145, #16120, #22715 ),
 ( #41510, #32537, #3370 ),
 ( #15704, #5736, #18689 ),
 ( #35116, #28709, #36387 ),
 ( #29560, #26782, #34178 ),
 ( #13579, #7203, #40004 ),
 ( #5004, #27767, #10795 ),
 ( #36169, #40778, #605 ) ),
 .UNSPECIFIED., .F., .F., .F. ) 
 B_SPLINE_SURFACE_WITH_KNOTS ( ( 4, 2, 2, 2, 2, 4 ),
 ( 3, 3 ),
 ( -3.945052844332828156E-19, 0.0001838632285168906972, 0.0003677264570337817739, 0.0007354529140675639814, 0.001103179371101346189, 0.001470905828135128397 ),
 ( 0.000000000000000000, 1.000000000000000000 ),
 .UNSPECIFIED. ) 
 GEOMETRIC_REPRESENTATION_ITEM ( )  RATIONAL_B_SPLINE_SURFACE ( (
 ( 1.000000000000000000, 0.7071067811865591191, 1.000000000000000000),
 ( 1.000000000000000000, 0.7071067811865591191, 1.000000000000000000),
 ( 1.000000000000000000, 0.7071067811865436870, 1.000000000000000000),
 ( 1.000000000000000000, 0.7071067811865436870, 1.000000000000000000),
 ( 1.000000000000000000, 0.7071067811865398012, 1.000000000000000000),
 ( 1.000000000000000000, 0.7071067811865398012, 1.000000000000000000),
 ( 1.000000000000000000, 0.7071067811865398012, 1.000000000000000000),
 ( 1.000000000000000000, 0.7071067811865398012, 1.000000000000000000),
 ( 1.000000000000000000, 0.7071067811865514585, 1.000000000000000000),
 ( 1.000000000000000000, 0.7071067811865514585, 1.000000000000000000),
 ( 1.000000000000000000, 0.7071067811865475727, 1.000000000000000000),
 ( 1.000000000000000000, 0.7071067811865475727, 1.000000000000000000) ) ) 
 REPRESENTATION_ITEM ( '' )  SURFACE ( )  );
#31900=B_SPLINE_CURVE_WITH_KNOTS ( 'NONE', 3,
 ( #31955, #19571, #9787, #32164, #12570, #15959 ),
 .UNSPECIFIED., .F., .F.,
 ( 4, 2, 4 ),
 ( 0.0007477044786394815333, 0.001108740074962825213, 0.001469775671286169001 ),
 .UNSPECIFIED. ) ;
#31923=LINE ( 'NONE', #12945, #27496 ) ;
#31928=CARTESIAN_POINT ( 'NONE',  ( 5.177913976931214357, 57.15000000000004832, 5.372099999999999653 ) ) ;
#31929=CARTESIAN_POINT ( 'NONE',  ( 14.73199999999999932, 12.96416000000000146, 0.000000000000000000 ) ) ;
#31934=AXIS2_PLACEMENT_3D ( 'NONE', #34110, #40709, #12144 ) ;
#31936=CARTESIAN_POINT ( 'NONE',  ( -10.45888906141547992, 56.51499999999998636, 4.393716635381797353 ) ) ;
#31940=DIRECTION ( 'NONE',  ( -1.000000000000000000, 9.563967653961371147E-17, 0.000000000000000000 ) ) ;
#31942=VERTEX_POINT ( 'NONE', #3634 ) ;
#31949=FACE_OUTER_BOUND ( 'NONE', #33455, .T. ) ;
#31955=CARTESIAN_POINT ( 'NONE',  ( 5.348924234570989533, 56.51499999999999346, -4.492130288940734850 ) ) ;
#31964=ORIENTED_EDGE ( 'NONE', *, *, #4603, .T. ) ;
#31975=DIRECTION ( 'NONE',  ( 1.000000000000000000, 2.185478394931408997E-15, 0.000000000000000000 ) ) ;
#31982=CARTESIAN_POINT ( 'NONE',  ( 17.14499999999999957, 71.11999999999999034, 5.016499999999999737 ) ) ;
#31999=DIRECTION ( 'NONE',  ( 6.353134868986659519E-16, -1.000000000000000000, 0.000000000000000000 ) ) ;
#32009=VECTOR ( 'NONE', #32119, 1000.000000000000000 ) ;
#32024=ORIENTED_EDGE ( 'NONE', *, *, #24223, .F. ) ;
#32030=EDGE_CURVE ( 'NONE', #35273, #40327, #7024, .T. ) ;
#32035=VECTOR ( 'NONE', #2108, 999.9999999999998863 ) ;
#32045=CARTESIAN_POINT ( 'NONE',  ( -5.475330206976889436, 77.01756249999996840, -5.107412922131463695 ) ) ;
#32076=AXIS2_PLACEMENT_3D ( 'NONE', #11319, #37516, #18122 ) ;
#32087=CARTESIAN_POINT ( 'NONE',  ( -5.177913976931285411, 57.14999999999998437, 5.372100000000002318 ) ) ;
#32109=VERTEX_POINT ( 'NONE', #14446 ) ;
#32113=CARTESIAN_POINT ( 'NONE',  ( -13.46199999999999264, 17.14499999999999957, 0.000000000000000000 ) ) ;
#32119=DIRECTION ( 'NONE',  ( -6.353134868986659519E-16, 1.000000000000000000, -0.000000000000000000 ) ) ;
#32125=VERTEX_POINT ( 'NONE', #4898 ) ;
#32134=FACE_OUTER_BOUND ( 'NONE', #17961, .T. ) ;
#32140=( BOUNDED_CURVE ( )  B_SPLINE_CURVE ( 3, ( #39430, #19809, #38794, #26638 ),
 .UNSPECIFIED., .F., .T. ) 
 B_SPLINE_CURVE_WITH_KNOTS ( ( 4, 4 ),
 ( 1.570796326794896558, 3.141592653589793116 ),
 .UNSPECIFIED. ) 
 CURVE ( )  GEOMETRIC_REPRESENTATION_ITEM ( )  RATIONAL_B_SPLINE_CURVE ( ( 1.000000000000000000, 0.8047378541243649375, 0.8047378541243649375, 1.000000000000000000 ) ) 
 REPRESENTATION_ITEM ( '' )  );
#32148=ADVANCED_FACE ( 'NONE', ( #4269 ), #26246, .T. ) ;
#32151=CARTESIAN_POINT ( 'NONE',  ( -17.14499999999999957, 71.11999999999999034, 5.016499999999999737 ) ) ;
#32159=CARTESIAN_POINT ( 'NONE',  ( 10.92199999999999704, 57.14999999999999858, 4.381499999999999950 ) ) ;
#32164=CARTESIAN_POINT ( 'NONE',  ( 5.817719362921480730, 56.51499999999997925, -4.384519708708640273 ) ) ;
#32167=EDGE_LOOP ( 'NONE', ( #14669, #30187, #16347, #2779 ) ) ;
#32172=AXIS2_PLACEMENT_3D ( 'NONE', #4456, #30620, #26804 ) ;
#32175=ORIENTED_EDGE ( 'NONE', *, *, #33529, .F. ) ;
#32176=VECTOR ( 'NONE', #26000, 1000.000000000000227 ) ;
#32177=EDGE_CURVE ( 'NONE', #22529, #21064, #14654, .T. ) ;
#32183=DIRECTION ( 'NONE',  ( 0.000000000000000000, 1.000000000000000000, 0.000000000000000000 ) ) ;
#32192=DIRECTION ( 'NONE',  ( -1.000000000000000000, 0.000000000000000000, 0.000000000000000000 ) ) ;
#32193=CIRCLE ( 'NONE', #4333, 0.6350000000000001199 ) ;
#32196=DIRECTION ( 'NONE',  ( 0.000000000000000000, 0.000000000000000000, -1.000000000000000000 ) ) ;
#32219=ORIENTED_EDGE ( 'NONE', *, *, #15810, .F. ) ;
#32220=CARTESIAN_POINT ( 'NONE',  ( 6.059261036834384662, 88.73331249999999670, 5.016499999999999737 ) ) ;
#32235=CARTESIAN_POINT ( 'NONE',  ( -3.590474171207809651E-14, 56.51499999999999346, 0.000000000000000000 ) ) ;
#32240=VERTEX_POINT ( 'NONE', #23613 ) ;
#32255=DIRECTION ( 'NONE',  ( 6.353134868986659519E-16, -1.000000000000000000, 0.000000000000000000 ) ) ;
#32262=DIRECTION ( 'NONE',  ( -9.627370216492862708E-17, -1.000000000000000000, 0.000000000000000000 ) ) ;
#32284=ORIENTED_EDGE ( 'NONE', *, *, #12352, .F. ) ;
#32295=CARTESIAN_POINT ( 'NONE',  ( 1.172031118611134874E-15, 12.17394877578616885, 0.000000000000000000 ) ) ;
#32300=LINE ( 'NONE', #31881, #37519 ) ;
#32314=CARTESIAN_POINT ( 'NONE',  ( 6.059261036834405978, 56.81853847168531502, -4.948064083792231393 ) ) ;
#32317=ORIENTED_EDGE ( 'NONE', *, *, #19110, .T. ) ;
#32327=CARTESIAN_POINT ( 'NONE',  ( 5.224239059777379346, 56.51499999999816737, 5.327449085207758728 ) ) ;
#32346=CARTESIAN_POINT ( 'NONE',  ( -6.059261036834472591, 56.51499999999997925, -4.381499999999997286 ) ) ;
#32350=EDGE_CURVE ( 'NONE', #18118, #4948, #2110, .T. ) ;
#32351=VERTEX_POINT ( 'NONE', #5735 ) ;
#32355=FACE_OUTER_BOUND ( 'NONE', #17179, .T. ) ;
#32356=B_SPLINE_SURFACE_WITH_KNOTS ( 'NONE', 5, 3, ( 
 ( #5870, #31837, #28851, #25651 ),
 ( #6282, #2467, #15429, #6077 ),
 ( #19253, #28218, #8626, #15634 ),
 ( #28639, #38449, #12458, #12026 ),
 ( #41650, #32045, #2882, #25452 ),
 ( #25018, #41864, #9265, #22224 ),
 ( #38020, #21589, #8841, #29054 ),
 ( #38239, #21804, #18622, #25235 ) ),
 .UNSPECIFIED., .F., .F., .F.,
 ( 6, 2, 6 ),
 ( 4, 4 ),
 ( 0.000000000000000000, 0.5000000000000000000, 1.000000000000000000 ),
 ( -0.002373312499999995218, 0.03277393749999999578 ),
 .UNSPECIFIED. ) ;
#32365=DIRECTION ( 'NONE',  ( -1.000000000000000000, 0.000000000000000000, 0.000000000000000000 ) ) ;
#32375=DIRECTION ( 'NONE',  ( -6.353134868986659519E-16, 1.000000000000000000, 0.000000000000000000 ) ) ;
#32395=ORIENTED_EDGE ( 'NONE', *, *, #32611, .F. ) ;
#32397=( BOUNDED_SURFACE ( )  B_SPLINE_SURFACE ( 3, 2, ( 
 ( #10871, #7065, #23859 ),
 ( #33472, #20029, #23642 ),
 ( #3878, #13862, #39864 ),
 ( #29843, #36664, #681 ),
 ( #13653, #7485, #26643 ),
 ( #4302, #14477, #37700 ),
 ( #37483, #11492, #8522 ),
 ( #18296, #8308, #24478 ),
 ( #33889, #40698, #34099 ),
 ( #24908, #27690, #31295 ) ),
 .UNSPECIFIED., .F., .F., .T. ) 
 B_SPLINE_SURFACE_WITH_KNOTS ( ( 4, 2, 2, 2, 4 ),
 ( 3, 3 ),
 ( -8.881784197001252323E-16, 0.3926990816987235844, 0.7853981633974480570, 1.178097245096172418, 1.570796326794897002 ),
 ( 0.000000000000000000, 1.000000000000000000 ),
 .UNSPECIFIED. ) 
 GEOMETRIC_REPRESENTATION_ITEM ( )  RATIONAL_B_SPLINE_SURFACE ( (
 ( 1.000000000000000000, 0.7572803591334833495, 1.000000000000000000),
 ( 1.000000000000000000, 0.7572851909592280828, 1.000000000000000000),
 ( 1.000000000000000000, 0.7560206254140621196, 1.000000000000000000),
 ( 1.000000000000000000, 0.7511365686956649190, 1.000000000000000000),
 ( 1.000000000000000000, 0.7475127447245452084, 1.000000000000000000),
 ( 1.000000000000000000, 0.7383589052087454752, 1.000000000000000000),
 ( 1.000000000000000000, 0.7328301610706697833, 1.000000000000000000),
 ( 1.000000000000000000, 0.7206031636699079534, 1.000000000000000000),
 ( 1.000000000000000000, 0.7139102541741279007, 1.000000000000000000),
 ( 1.000000000000000000, 0.7071067811865475727, 1.000000000000000000) ) ) 
 REPRESENTATION_ITEM ( '' )  SURFACE ( )  );
#32399=CIRCLE ( 'NONE', #18794, 0.6350000000000001199 ) ;
#32401=VECTOR ( 'NONE', #16465, 1000.000000000000000 ) ;
#32437=DIRECTION ( 'NONE',  ( -0.000000000000000000, -0.000000000000000000, -1.000000000000000000 ) ) ;
#32451=AXIS2_PLACEMENT_3D ( 'NONE', #21947, #25374, #31337 ) ;
#32469=CARTESIAN_POINT ( 'NONE',  ( 7.461249999999945537, 85.80437499999999318, 0.000000000000000000 ) ) ;
#32476=ORIENTED_EDGE ( 'NONE', *, *, #41215, .T. ) ;
#32477=FACE_OUTER_BOUND ( 'NONE', #23896, .T. ) ;
#32488=CARTESIAN_POINT ( 'NONE',  ( -3.630816577625874595E-14, 57.14999999999999147, 0.000000000000000000 ) ) ;
#32502=CIRCLE ( 'NONE', #3931, 7.461249999999999716 ) ;
#32504=ORIENTED_EDGE ( 'NONE', *, *, #11519, .T. ) ;
#32507=PLANE ( 'NONE',  #3657 ) ;
#32509=ORIENTED_EDGE ( 'NONE', *, *, #7929, .T. ) ;
#32512=CARTESIAN_POINT ( 'NONE',  ( -9.638062024671791406, 56.51499999999998636, 3.341163682266966022E-16 ) ) ;
#32523=CARTESIAN_POINT ( 'NONE',  ( -18.35410564743290607, 77.35382415001784295, -1.904999999999999583 ) ) ;
#32532=PLANE ( 'NONE',  #1357 ) ;
#32537=CARTESIAN_POINT ( 'NONE',  ( 5.449227423685711891, 56.51499999999995794, 5.145694933557973805 ) ) ;
#32554=CARTESIAN_POINT ( 'NONE',  ( -4.918266948219002899, 56.51499999999997215, -4.748921713023556812 ) ) ;
#32556=CARTESIAN_POINT ( 'NONE',  ( 5.299459906814694143, 78.93540349268872092, 5.255323016343538711 ) ) ;
#32559=CARTESIAN_POINT ( 'NONE',  ( -6.059261036834476144, 56.51499999999998636, 4.381499999999999950 ) ) ;
#32573=DIRECTION ( 'NONE',  ( 9.627370216492862708E-17, 1.000000000000000000, -0.000000000000000000 ) ) ;
#32579=DIRECTION ( 'NONE',  ( -9.627370216492862708E-17, -1.000000000000000000, 0.000000000000000000 ) ) ;
#32592=VERTEX_POINT ( 'NONE', #29122 ) ;
#32595=SHAPE_REPRESENTATION_RELATIONSHIP ( 'NONE' , 'NONE' ,  #11484, #21408 ) ;
#32606=DIRECTION ( 'NONE',  ( -0.000000000000000000, -0.000000000000000000, -1.000000000000000000 ) ) ;
#32611=EDGE_CURVE ( 'NONE', #37685, #27491, #32974, .T. ) ;
#32612=CARTESIAN_POINT ( 'NONE',  ( -13.51785991797444098, 17.08228783296376108, 5.016499999999999737 ) ) ;
#32634=TOROIDAL_SURFACE ( 'NONE', #37404, 15.36699999999999555, 0.6350000000000000089 ) ;
#32635=EDGE_LOOP ( 'NONE', ( #5370, #29822, #22249, #30748, #15358, #41459, #23232 ) ) ;
#32664=CARTESIAN_POINT ( 'NONE',  ( -17.14499999999999957, 71.11999999999999034, -5.016499999999999737 ) ) ;
#32679=CARTESIAN_POINT ( 'NONE',  ( -11.65115770210962687, 16.51000000000000156, 4.908176479697702099 ) ) ;
#32682=CARTESIAN_POINT ( 'NONE',  ( -9.094996104468901166, 78.64197151092922411, -5.392902600000144986 ) ) ;
#32686=EDGE_CURVE ( 'NONE', #18659, #329, #29359, .T. ) ;
#32690=VERTEX_POINT ( 'NONE', #9849 ) ;
#32703=FACE_OUTER_BOUND ( 'NONE', #27592, .T. ) ;
#32720=ORIENTED_EDGE ( 'NONE', *, *, #39685, .T. ) ;
#32745=VECTOR ( 'NONE', #2391, 1000.000000000000000 ) ;
#32761=VERTEX_POINT ( 'NONE', #26882 ) ;
#32771=CIRCLE ( 'NONE', #25940, 6.350000000000004974 ) ;
#32787=PLANE ( 'NONE',  #2952 ) ;
#32794=CYLINDRICAL_SURFACE ( 'NONE', #7440, 12.69999999999999751 ) ;
#32797=( NAMED_UNIT ( * ) PLANE_ANGLE_UNIT ( ) SI_UNIT ( $, .RADIAN. ) );
#32814=PRODUCT_CONTEXT ( 'NONE', #30877, 'mechanical' ) ;
#32826=CARTESIAN_POINT ( 'NONE',  ( 17.14499999999999957, 71.11999999999999034, 5.016499999999999737 ) ) ;
#32833=DIRECTION ( 'NONE',  ( -1.000000000000000000, 0.000000000000000000, 0.000000000000000000 ) ) ;
#32845=CARTESIAN_POINT ( 'NONE',  ( 13.85159022459153988, 12.96416000000000146, -5.016499999999999737 ) ) ;
#32849=AXIS2_PLACEMENT_3D ( 'NONE', #40232, #11027, #24008 ) ;
#32850=CARTESIAN_POINT ( 'NONE',  ( -12.21488373879589240, 71.11999999999999034, -5.016499999999999737 ) ) ;
#32853=ORIENTED_EDGE ( 'NONE', *, *, #33432, .F. ) ;
#32895=CARTESIAN_POINT ( 'NONE',  ( -5.177913976931289852, 65.30181249999996851, 5.372100000000007647 ) ) ;
#32914=DIRECTION ( 'NONE',  ( -6.353134868986659519E-16, 1.000000000000000000, -0.000000000000000000 ) ) ;
#32918=CARTESIAN_POINT ( 'NONE',  ( 1.248107678658480997E-15, 12.96416000000000146, 0.000000000000000000 ) ) ;
#32952=DIRECTION ( 'NONE',  ( 0.8138664877804109299, -0.5810519254489895369, 0.000000000000000000 ) ) ;
#32974=LINE ( 'NONE', #9950, #32009 ) ;
#32989=CARTESIAN_POINT ( 'NONE',  ( -20.83467972660109169, 65.95194780259438971, -5.016499999999999737 ) ) ;
#33002=CARTESIAN_POINT ( 'NONE',  ( -5.237865101059587580, 78.94033958618261693, -5.314315937239334708 ) ) ;
#33010=FACE_OUTER_BOUND ( 'NONE', #18299, .T. ) ;
#33020=DIRECTION ( 'NONE',  ( 9.627370216492862708E-17, 1.000000000000000000, -0.000000000000000000 ) ) ;
#33026=VERTEX_POINT ( 'NONE', #40317 ) ;
#33043=CARTESIAN_POINT ( 'NONE',  ( -17.14499999999999957, 71.11999999999999034, 5.016499999999999737 ) ) ;
#33047=PLANE ( 'NONE',  #29156 ) ;
#33055=CARTESIAN_POINT ( 'NONE',  ( -5.892673590944178308, 78.88814725119665638, 5.017439957471214740 ) ) ;
#33056=FACE_BOUND ( 'NONE', #27176, .T. ) ;
#33068=ORIENTED_EDGE ( 'NONE', *, *, #31099, .F. ) ;
#33076=DIRECTION ( 'NONE',  ( -9.627370216492862708E-17, -1.000000000000000000, 0.000000000000000000 ) ) ;
#33084=CARTESIAN_POINT ( 'NONE',  ( -5.424023212060650856, 78.92586886208859198, 5.134886908577998454 ) ) ;
#33118=VERTEX_POINT ( 'NONE', #40931 ) ;
#33139=VECTOR ( 'NONE', #27723, 1000.000000000000114 ) ;
#33150=CARTESIAN_POINT ( 'NONE',  ( -11.41714695485569919, 57.14999999999997726, 5.016500000000000625 ) ) ;
#33167=ORIENTED_EDGE ( 'NONE', *, *, #10027, .T. ) ;
#33179=CARTESIAN_POINT ( 'NONE',  ( 6.057513928997569685, 57.78500000000000369, 1.904999999999996030 ) ) ;
#33225=EDGE_CURVE ( 'NONE', #21005, #22572, #8338, .T. ) ;
#33228=DIRECTION ( 'NONE',  ( 1.224646799147353207E-16, 7.780346281855952181E-32, 1.000000000000000000 ) ) ;
#33239=EDGE_LOOP ( 'NONE', ( #10597, #10727, #19645, #37197 ) ) ;
#33252=CARTESIAN_POINT ( 'NONE',  ( 12.21488373879589240, 17.14499999999999957, -4.381499999999999950 ) ) ;
#33259=AXIS2_PLACEMENT_3D ( 'NONE', #15234, #18638, #34421 ) ;
#33264=ORIENTED_EDGE ( 'NONE', *, *, #38528, .T. ) ;
#33268=CARTESIAN_POINT ( 'NONE',  ( 6.349999999999963229, 57.78500000000000369, 0.000000000000000000 ) ) ;
#33292=VECTOR ( 'NONE', #20713, 1000.000000000000114 ) ;
#33294=CLOSED_SHELL ( 'NONE', ( #35232, #9267, #23652, #8998, #4644, #12567, #12595, #4214, #920, #23538, #3678, #26093, #5885, #36559, #2767, #306, #12100, #16975, #29731, #12360, #36744, #25533, #12412, #21950, #27841, #5168, #33672, #32148, #37116, #28524, #34175, #10285, #8168, #25608, #14441, #27628, #28689, #10287, #24367, #6545, #14803, #29197, #41210, #3379, #21687, #934, #23732, #17771, #16466, #38714, #22743, #36229, #19568, #29533, #8225, #12331, #31040, #13648, #17592, #39749, #1910, #38112, #29796, #17824, #16041, #3806, #14512, #24494, #19593, #9910, #8901, #5939, #12695, #22913, #21643, #18773, #14215, #20166, #23238, #11734, #35031, #1727, #18651, #15668, #884, #14166, #17830, #8261, #16468, #42011, #21967, #12066, #38905, #14678, #24762, #22999, #23691, #39348, #14311, #1132, #17555, #36361, #31620, #28133, #9811, #41422, #14680, #28186, #14090, #15695, #23530, #3225, #4300, #34697, #19074 ) ) ;
#33297=ORIENTED_EDGE ( 'NONE', *, *, #36608, .F. ) ;
#33300=ORIENTED_EDGE ( 'NONE', *, *, #2888, .T. ) ;
#33316=CARTESIAN_POINT ( 'NONE',  ( -5.475330206976867231, 53.58606250000000415, 5.107412922131463695 ) ) ;
#33336=CARTESIAN_POINT ( 'NONE',  ( -7.213960532367465817, 78.77618639008778700, -1.904999999999999583 ) ) ;
#33368=ORIENTED_EDGE ( 'NONE', *, *, #5064, .F. ) ;
#33371=ORIENTED_EDGE ( 'NONE', *, *, #27169, .T. ) ;
#33382=CARTESIAN_POINT ( 'NONE',  ( 10.92199999999999704, 12.96416000000000146, 0.000000000000000000 ) ) ;
#33398=AXIS2_PLACEMENT_3D ( 'NONE', #1514, #14471, #31501 ) ;
#33399=DIRECTION ( 'NONE',  ( -6.353134868986659519E-16, 1.000000000000000000, 0.000000000000000000 ) ) ;
#33428=AXIS2_PLACEMENT_3D ( 'NONE', #25693, #22683, #42116 ) ;
#33432=EDGE_CURVE ( 'NONE', #22572, #3641, #28136, .T. ) ;
#33436=CARTESIAN_POINT ( 'NONE',  ( 14.39766717389552220, 60.87500489999898434, 1.904999999999990257 ) ) ;
#33448=ORIENTED_EDGE ( 'NONE', *, *, #11494, .F. ) ;
#33455=EDGE_LOOP ( 'NONE', ( #11223, #7646, #36472, #21573, #41359, #13101, #38662, #11160 ) ) ;
#33465=AXIS2_PLACEMENT_3D ( 'NONE', #19189, #32196, #3030 ) ;
#33472=CARTESIAN_POINT ( 'NONE',  ( 12.21488373878702127, 55.49440886859300548, 5.016499999999999737 ) ) ;
#33492=ORIENTED_EDGE ( 'NONE', *, *, #3776, .F. ) ;
#33497=VERTEX_POINT ( 'NONE', #5998 ) ;
#33510=CARTESIAN_POINT ( 'NONE',  ( 10.79307885933854294, 57.10041794475097987, -5.016500000000000625 ) ) ;
#33529=EDGE_CURVE ( 'NONE', #40534, #20298, #9185, .T. ) ;
#33535=ORIENTED_EDGE ( 'NONE', *, *, #26947, .F. ) ;
#33547=B_SPLINE_CURVE_WITH_KNOTS ( 'NONE', 3,
 ( #23866, #26864, #896, #40083, #36885, #7703, #39872, #13871, #20242, #23218, #30058, #23432, #4309, #14274, #17056, #20666, #479, #7073, #33690, #10463, #16850, #33055, #10879, #29850 ),
 .UNSPECIFIED., .F., .F.,
 ( 4, 2, 2, 2, 1, 2, 2, 2, 2, 1, 2, 2, 4 ),
 ( 0.000000000000000000, 0.2499999999999849565, 0.3749999999999771849, 0.4374999999999723554, 0.4687499999999691358, 0.4843749999999673039, 0.4999999999999654721, 0.6249999999999718003, 0.6874999999999765743, 0.7187499999999787947, 0.7343749999999799050, 0.7499999999999809042, 1.000000000000000000 ),
 .UNSPECIFIED. ) ;
#33552=CARTESIAN_POINT ( 'NONE',  ( 10.38331224698210242, 57.14999999999999858, 5.016499999999999737 ) ) ;
#33580=AXIS2_PLACEMENT_3D ( 'NONE', #6683, #19864, #38644 ) ;
#33592=DIRECTION ( 'NONE',  ( -6.353134868986659519E-16, 1.000000000000000000, 0.000000000000000000 ) ) ;
#33598=PLANE ( 'NONE',  #25162 ) ;
#33599=VERTEX_POINT ( 'NONE', #16051 ) ;
#33605=AXIS2_PLACEMENT_3D ( 'NONE', #798, #10367, #4629 ) ;
#33617=EDGE_CURVE ( 'NONE', #19469, #27131, #35049, .T. ) ;
#33633=EDGE_CURVE ( 'NONE', #14016, #4305, #19039, .T. ) ;
#33667=EDGE_LOOP ( 'NONE', ( #10169, #16390, #5452, #22192 ) ) ;
#33672=ADVANCED_FACE ( 'NONE', ( #5665 ), #32356, .T. ) ;
#33678=EDGE_CURVE ( 'NONE', #16922, #700, #40571, .T. ) ;
#33683=DIRECTION ( 'NONE',  ( -0.000000000000000000, -0.000000000000000000, -1.000000000000000000 ) ) ;
#33686=EDGE_LOOP ( 'NONE', ( #4228, #31964 ) ) ;
#33690=CARTESIAN_POINT ( 'NONE',  ( -5.787341484272856107, 78.89667267365574332, 5.030122981225376932 ) ) ;
#33701=AXIS2_PLACEMENT_3D ( 'NONE', #40143, #10935, #29601 ) ;
#33703=ORIENTED_EDGE ( 'NONE', *, *, #14042, .T. ) ;
#33710=ORIENTED_EDGE ( 'NONE', *, *, #16668, .F. ) ;
#33718=DIRECTION ( 'NONE',  ( 0.000000000000000000, 1.000000000000000000, 0.000000000000000000 ) ) ;
#33723=EDGE_CURVE ( 'NONE', #20581, #40888, #35123, .T. ) ;
#33725=EDGE_CURVE ( 'NONE', #42131, #37617, #7903, .T. ) ;
#33780=FACE_OUTER_BOUND ( 'NONE', #15839, .T. ) ;
#33789=CARTESIAN_POINT ( 'NONE',  ( 14.73199999999999932, 57.78500000000000369, 4.848162602465631106E-15 ) ) ;
#33801=CARTESIAN_POINT ( 'NONE',  ( -7.017589760824602507, 78.79342665089201603, -2.556811674275342394 ) ) ;
#33803=VERTEX_POINT ( 'NONE', #33992 ) ;
#33813=AXIS2_PLACEMENT_3D ( 'NONE', #40433, #17611, #30612 ) ;
#33827=EDGE_CURVE ( 'NONE', #1007, #11738, #27996, .T. ) ;
#33841=AXIS2_PLACEMENT_3D ( 'NONE', #8108, #21082, #14275 ) ;
#33859=CARTESIAN_POINT ( 'NONE',  ( 6.059261036834406866, 53.58606249999999704, -5.016499999999999737 ) ) ;
#33875=B_SPLINE_CURVE_WITH_KNOTS ( 'NONE', 3,
 ( #25141, #38145, #5778, #7548, #31743, #28548 ),
 .UNSPECIFIED., .F., .F.,
 ( 4, 2, 4 ),
 ( -7.295512689534840788E-06, 0.0003601880853872708229, 0.0007276716834640765052 ),
 .UNSPECIFIED. ) ;
#33884=CARTESIAN_POINT ( 'NONE',  ( -13.85159022459153988, 12.96416000000000146, 5.016499999999999737 ) ) ;
#33889=CARTESIAN_POINT ( 'NONE',  ( 10.54112285291074969, 57.14999999999387370, 5.016499999999999737 ) ) ;
#33925=EDGE_CURVE ( 'NONE', #24827, #25936, #31188, .T. ) ;
#33928=ORIENTED_EDGE ( 'NONE', *, *, #27913, .T. ) ;
#33931=CIRCLE ( 'NONE', #22328, 2.540000000000000480 ) ;
#33932=CARTESIAN_POINT ( 'NONE',  ( 11.66725022230187214, 55.42194143536249840, -5.016499999999354031 ) ) ;
#33941=CARTESIAN_POINT ( 'NONE',  ( -11.62920297224754762, 55.59919541885980721, 5.016499999999892268 ) ) ;
#33947=CARTESIAN_POINT ( 'NONE',  ( 14.60500000000000043, 71.11999999999999034, 1.904999999999990701 ) ) ;
#33949=CARTESIAN_POINT ( 'NONE',  ( -5.177913976931286300, 57.14999999999999858, 5.372100000000003206 ) ) ;
#33970=CARTESIAN_POINT ( 'NONE',  ( 6.059261036834406866, 56.81853847168529370, 4.948064083792229617 ) ) ;
#33978=EDGE_LOOP ( 'NONE', ( #36264, #29934, #42078, #7504 ) ) ;
#33981=FACE_OUTER_BOUND ( 'NONE', #35640, .T. ) ;
#33987=CIRCLE ( 'NONE', #26486, 0.5556250000000014788 ) ;
#33992=CARTESIAN_POINT ( 'NONE',  ( -19.68500000000000227, 71.11999999999999034, -5.016499999999999737 ) ) ;
#34016=AXIS2_PLACEMENT_3D ( 'NONE', #29410, #39215, #464 ) ;
#34036=LINE ( 'NONE', #31028, #18820 ) ;
#34041=CARTESIAN_POINT ( 'NONE',  ( -13.85159022459153988, 12.96416000000000146, -5.016499999999999737 ) ) ;
#34051=ORIENTED_EDGE ( 'NONE', *, *, #8932, .F. ) ;
#34053=EDGE_CURVE ( 'NONE', #35130, #5873, #19452, .T. ) ;
#34065=DIRECTION ( 'NONE',  ( -6.353134868986659519E-16, 1.000000000000000000, 0.000000000000000000 ) ) ;
#34099=CARTESIAN_POINT ( 'NONE',  ( 10.45888906141538399, 56.51500000000000057, 4.393716635381806235 ) ) ;
#34107=CARTESIAN_POINT ( 'NONE',  ( -12.16475753114696978, 55.74362973025101553, -5.016499999999999737 ) ) ;
#34110=CARTESIAN_POINT ( 'NONE',  ( -3.630816577625875226E-14, 57.14999999999999147, 0.000000000000000000 ) ) ;
#34139=DIRECTION ( 'NONE',  ( 1.000000000000000000, -1.177520686924251719E-16, 0.000000000000000000 ) ) ;
#34158=DIRECTION ( 'NONE',  ( -1.000000000000000000, 0.000000000000000000, 0.000000000000000000 ) ) ;
#34160=DIRECTION ( 'NONE',  ( -1.000000000000000000, 0.000000000000000000, 0.000000000000000000 ) ) ;
#34175=ADVANCED_FACE ( 'NONE', ( #42064 ), #34445, .T. ) ;
#34178=CARTESIAN_POINT ( 'NONE',  ( 5.706393392231229988, 57.14999999999913882, 5.041882957777255037 ) ) ;
#34184=AXIS2_PLACEMENT_3D ( 'NONE', #29005, #6859, #26018 ) ;
#34197=EDGE_CURVE ( 'NONE', #1422, #6797, #15626, .T. ) ;
#34216=CARTESIAN_POINT ( 'NONE',  ( 14.73199999999999754, 17.14499999999999957, 1.804149664503880250E-15 ) ) ;
#34222=CONICAL_SURFACE ( 'NONE', #32849, 12.69999999999999751, 0.7853981633974471688 ) ;
#34223=ORIENTED_EDGE ( 'NONE', *, *, #30555, .F. ) ;
#34240=CARTESIAN_POINT ( 'NONE',  ( 5.249640227149889427, 56.51499999999963819, 4.563681476173430340 ) ) ;
#34243=DIRECTION ( 'NONE',  ( 0.000000000000000000, 0.000000000000000000, 1.000000000000000000 ) ) ;
#34245=FACE_OUTER_BOUND ( 'NONE', #28520, .T. ) ;
#34253=CARTESIAN_POINT ( 'NONE',  ( 5.706177858098580913, 57.14999999999916724, -5.041924732081959348 ) ) ;
#34279=DIRECTION ( 'NONE',  ( 0.000000000000000000, 1.000000000000000000, 0.000000000000000000 ) ) ;
#34298=ORIENTED_EDGE ( 'NONE', *, *, #22871, .T. ) ;
#34346=ORIENTED_EDGE ( 'NONE', *, *, #40277, .F. ) ;
#34348=CARTESIAN_POINT ( 'NONE',  ( 11.97180806971946332, 56.20439414706017089, -5.016500000000000625 ) ) ;
#34380=CARTESIAN_POINT ( 'NONE',  ( -13.85159022459153988, 12.96416000000000146, -5.016499999999999737 ) ) ;
#34399=DIRECTION ( 'NONE',  ( 0.8138664877804109299, 0.5810519254489895369, 0.000000000000000000 ) ) ;
#34408=ORIENTED_EDGE ( 'NONE', *, *, #29800, .F. ) ;
#34418=CARTESIAN_POINT ( 'NONE',  ( 14.39766717389552042, 60.02151067229126369, -1.904999999999999583 ) ) ;
#34421=DIRECTION ( 'NONE',  ( 1.000000000000000000, 0.000000000000000000, -5.975917486140574681E-16 ) ) ;
#34445=TOROIDAL_SURFACE ( 'NONE', #38521, 6.905624999999998792, 0.5556250000000014788 ) ;
#34446=ORIENTED_EDGE ( 'NONE', *, *, #32350, .T. ) ;
#34457=DIRECTION ( 'NONE',  ( 1.000000000000000000, -9.627370216492862708E-17, 0.000000000000000000 ) ) ;
#34476=CARTESIAN_POINT ( 'NONE',  ( 5.424023212060550492, 78.92586886208859198, -5.134886908577998454 ) ) ;
#34495=ORIENTED_EDGE ( 'NONE', *, *, #20228, .T. ) ;
#34496=VECTOR ( 'NONE', #31550, 1000.000000000000000 ) ;
#34507=CARTESIAN_POINT ( 'NONE',  ( 5.938381009910428610, 56.51499999999999346, 4.381499999999999062 ) ) ;
#34511=DIRECTION ( 'NONE',  ( 9.627370216492862708E-17, 1.000000000000000000, -0.000000000000000000 ) ) ;
#34514=CARTESIAN_POINT ( 'NONE',  ( -6.059261036834476144, 57.14999999999999858, -5.016499999999999737 ) ) ;
#34524=CARTESIAN_POINT ( 'NONE',  ( -11.66725022230187037, 55.42194143536166706, -5.016499999999783910 ) ) ;
#34526=AXIS2_PLACEMENT_3D ( 'NONE', #32488, #22660, #41457 ) ;
#34545=ORIENTED_EDGE ( 'NONE', *, *, #30069, .F. ) ;
#34580=ORIENTED_EDGE ( 'NONE', *, *, #5011, .T. ) ;
#34599=ORIENTED_EDGE ( 'NONE', *, *, #586, .T. ) ;
#34602=AXIS2_PLACEMENT_3D ( 'NONE', #29210, #25598, #53 ) ;
#34605=DIRECTION ( 'NONE',  ( -0.000000000000000000, -0.000000000000000000, -1.000000000000000000 ) ) ;
#34613=DIRECTION ( 'NONE',  ( 0.000000000000000000, 0.000000000000000000, 1.000000000000000000 ) ) ;
#34616=AXIS2_PLACEMENT_3D ( 'NONE', #10109, #35474, #36114 ) ;
#34650=VECTOR ( 'NONE', #39238, 1000.000000000000000 ) ;
#34652=CIRCLE ( 'NONE', #25787, 6.349999999999999645 ) ;
#34658=CARTESIAN_POINT ( 'NONE',  ( 1.650612623617701257E-15, 17.14499999999999957, 0.000000000000000000 ) ) ;
#34664=CARTESIAN_POINT ( 'NONE',  ( 5.936145915410036444, 56.51500000000000057, -4.381499802576882097 ) ) ;
#34666=CARTESIAN_POINT ( 'NONE',  ( 5.177913976931196594, 78.94499979771845233, 5.372100000000001430 ) ) ;
#34678=DIRECTION ( 'NONE',  ( 1.000000000000000000, -9.627370216492862708E-17, 0.000000000000000000 ) ) ;
#34682=CARTESIAN_POINT ( 'NONE',  ( -7.127785904777471870, 78.78377652171661794, 2.231330898844070987 ) ) ;
#34697=ADVANCED_FACE ( 'NONE', ( #23054 ), #21793, .T. ) ;
#34708=DIRECTION ( 'NONE',  ( 9.627370216492862708E-17, 1.000000000000000000, -0.000000000000000000 ) ) ;
#34719=CARTESIAN_POINT ( 'NONE',  ( -5.309060684617390516E-14, 83.56599999999998829, 0.000000000000000000 ) ) ;
#34730=CARTESIAN_POINT ( 'NONE',  ( 14.60500000000000043, 71.11999999999999034, 5.016499999999999737 ) ) ;
#34731=DIRECTION ( 'NONE',  ( 0.000000000000000000, 0.000000000000000000, 1.000000000000000000 ) ) ;
#34745=VECTOR ( 'NONE', #39444, 999.9999999999998863 ) ;
#34747=ORIENTED_EDGE ( 'NONE', *, *, #12874, .F. ) ;
#34749=CARTESIAN_POINT ( 'NONE',  ( 13.73816324777078890, 59.55066437026322745, 5.662797264199856073 ) ) ;
#34752=DIRECTION ( 'NONE',  ( 5.463695987328526437E-16, -1.000000000000000000, -1.672774450599033775E-31 ) ) ;
#34761=EDGE_CURVE ( 'NONE', #19019, #1397, #35972, .T. ) ;
#34762=VERTEX_POINT ( 'NONE', #19755 ) ;
#34782=CIRCLE ( 'NONE', #4874, 0.6350000000000001199 ) ;
#34785=CARTESIAN_POINT ( 'NONE',  ( 4.897655256226217446, 56.53910281269280347, -5.081330806033660608 ) ) ;
#34790=EDGE_LOOP ( 'NONE', ( #3339, #16383, #6059, #39051, #37589, #25730, #24717, #584 ) ) ;
#34837=FACE_OUTER_BOUND ( 'NONE', #18279, .T. ) ;
#34838=ORIENTED_EDGE ( 'NONE', *, *, #3434, .T. ) ;
#34843=CARTESIAN_POINT ( 'NONE',  ( 5.496588887047727745, 78.91991874857603761, -5.121802412194443654 ) ) ;
#34852=DIRECTION ( 'NONE',  ( 0.000000000000000000, -1.000000000000000000, -0.000000000000000000 ) ) ;
#34870=DIRECTION ( 'NONE',  ( -0.1469470846586743706, -9.335746474409589170E-17, -0.9891443546370348727 ) ) ;
#34872=AXIS2_PLACEMENT_3D ( 'NONE', #31525, #2369, #15327 ) ;
#34879=CARTESIAN_POINT ( 'NONE',  ( 4.737240446979628317, 56.51499999999997215, -4.914899999999988722 ) ) ;
#34883=CARTESIAN_POINT ( 'NONE',  ( -5.638141748386694907, 56.51500000000081769, 5.060111600421964617 ) ) ;
#34894=ORIENTED_EDGE ( 'NONE', *, *, #21122, .F. ) ;
#34903=CARTESIAN_POINT ( 'NONE',  ( -10.92199999999999704, 12.96416000000000146, 0.000000000000000000 ) ) ;
#34904=CARTESIAN_POINT ( 'NONE',  ( 5.256666791691227303, 57.14999999999997726, 5.296388421271908342 ) ) ;
#34918=ORIENTED_EDGE ( 'NONE', *, *, #16264, .F. ) ;
#34920=AXIS2_PLACEMENT_3D ( 'NONE', #6167, #35971, #19340 ) ;
#34925=VERTEX_POINT ( 'NONE', #9725 ) ;
#34932=DIRECTION ( 'NONE',  ( -0.000000000000000000, 0.000000000000000000, -1.000000000000000000 ) ) ;
#34935=CARTESIAN_POINT ( 'NONE',  ( 5.435468916198098022, 78.92497954178514874, 5.153742819108977358 ) ) ;
#34952=LINE ( 'NONE', #28545, #22580 ) ;
#34986=DIRECTION ( 'NONE',  ( -9.627370216492862708E-17, -1.000000000000000000, 0.000000000000000000 ) ) ;
#34988=CARTESIAN_POINT ( 'NONE',  ( -13.17422243436020857, 17.14500000000000668, 5.016499999999999737 ) ) ;
#35010=ORIENTED_EDGE ( 'NONE', *, *, #16531, .F. ) ;
#35031=ADVANCED_FACE ( 'NONE', ( #6964, #585 ), #25497, .F. ) ;
#35033=ORIENTED_EDGE ( 'NONE', *, *, #19302, .T. ) ;
#35049=LINE ( 'NONE', #35253, #24912 ) ;
#35053=VERTEX_POINT ( 'NONE', #30160 ) ;
#35095=CARTESIAN_POINT ( 'NONE',  ( 5.224225368397438451, 56.51500000000548596, -5.327462281792795906 ) ) ;
#35098=CARTESIAN_POINT ( 'NONE',  ( -5.511275327877945607, 57.14999999999955804, 5.111309965977547165 ) ) ;
#35116=CARTESIAN_POINT ( 'NONE',  ( 5.450291846086562586, 56.51499999999996504, 4.451173312910839286 ) ) ;
#35123=CIRCLE ( 'NONE', #10628, 14.73199999999999577 ) ;
#35130=VERTEX_POINT ( 'NONE', #1209 ) ;
#35133=CARTESIAN_POINT ( 'NONE',  ( 6.057513928997551922, 83.56599999999998829, -1.904999999999999805 ) ) ;
#35155=CARTESIAN_POINT ( 'NONE',  ( -5.664977208693890987, 57.14999999999997016, -5.033228321271210781 ) ) ;
#35158=DIRECTION ( 'NONE',  ( 0.9849462604886048966, 0.000000000000000000, -0.1728608224830406881 ) ) ;
#35178=AXIS2_PLACEMENT_3D ( 'NONE', #41051, #5484, #34243 ) ;
#35185=ORIENTED_EDGE ( 'NONE', *, *, #35461, .F. ) ;
#35196=CARTESIAN_POINT ( 'NONE',  ( 18.32410244842765934, 0.6349999999999984546, 2.244055341071511024E-15 ) ) ;
#35203=DIRECTION ( 'NONE',  ( -1.000000000000000000, -5.463695987328526437E-16, -0.000000000000000000 ) ) ;
#35207=DIRECTION ( 'NONE',  ( -0.000000000000000000, -0.000000000000000000, -1.000000000000000000 ) ) ;
#35213=CARTESIAN_POINT ( 'NONE',  ( 5.475330206976798841, 53.58606249999999704, 5.107412922131463695 ) ) ;
#35232=ADVANCED_FACE ( 'NONE', ( #36564 ), #5233, .T. ) ;
#35241=DIRECTION ( 'NONE',  ( 6.146657985744592735E-16, 3.905054717696927382E-31, 1.000000000000000000 ) ) ;
#35246=EDGE_CURVE ( 'NONE', #11189, #5419, #40186, .T. ) ;
#35253=CARTESIAN_POINT ( 'NONE',  ( -16.60960244842765832, 17.14499999999999957, 0.000000000000000000 ) ) ;
#35268=CARTESIAN_POINT ( 'NONE',  ( -17.68910244842765778, 3.329298639413090771E-15, 2.205172805198582110E-15 ) ) ;
#35272=CARTESIAN_POINT ( 'NONE',  ( 1.650612623617701257E-15, 17.14499999999999957, 0.000000000000000000 ) ) ;
#35273=VERTEX_POINT ( 'NONE', #7589 ) ;
#35292=AXIS2_PLACEMENT_3D ( 'NONE', #14741, #27951, #27743 ) ;
#35293=LINE ( 'NONE', #26115, #10300 ) ;
#35298=DIRECTION ( 'NONE',  ( -0.5810519254489896479, -0.8138664877804110409, 0.000000000000000000 ) ) ;
#35299=DIRECTION ( 'NONE',  ( 0.000000000000000000, 0.000000000000000000, -1.000000000000000000 ) ) ;
#35338=EDGE_CURVE ( 'NONE', #24583, #22830, #15428, .T. ) ;
#35348=VERTEX_POINT ( 'NONE', #27793 ) ;
#35360=CARTESIAN_POINT ( 'NONE',  ( 19.68500000000000227, 71.11999999999999034, 1.904999999999987592 ) ) ;
#35371=CIRCLE ( 'NONE', #12899, 13.46199999999999619 ) ;
#35375=( NAMED_UNIT ( * ) PLANE_ANGLE_UNIT ( ) SI_UNIT ( $, .RADIAN. ) );
#35381=CARTESIAN_POINT ( 'NONE',  ( 10.92199999999999704, 56.51500000000000057, -4.381499999999999950 ) ) ;
#35415=CARTESIAN_POINT ( 'NONE',  ( 5.871452009091292723, 88.73331249999999670, 5.016499999999999737 ) ) ;
#35417=DIRECTION ( 'NONE',  ( -0.1728608224830406603, 0.000000000000000000, -0.9849462604886047856 ) ) ;
#35430=DIRECTION ( 'NONE',  ( -6.353134868986659519E-16, 1.000000000000000000, 0.000000000000000000 ) ) ;
#35438=ORIENTED_EDGE ( 'NONE', *, *, #22158, .T. ) ;
#35443=EDGE_CURVE ( 'NONE', #9633, #3167, #2252, .T. ) ;
#35446=CARTESIAN_POINT ( 'NONE',  ( -1.915954025944994433E-14, 30.83083951148100255, 1.904999999999999805 ) ) ;
#35455=VECTOR ( 'NONE', #3871, 1000.000000000000114 ) ;
#35461=EDGE_CURVE ( 'NONE', #35130, #18118, #25852, .T. ) ;
#35466=ORIENTED_EDGE ( 'NONE', *, *, #23472, .F. ) ;
#35474=DIRECTION ( 'NONE',  ( -6.146657985744592735E-16, 3.905054717696928257E-31, 1.000000000000000000 ) ) ;
#35477=CARTESIAN_POINT ( 'NONE',  ( -13.46199999999999264, 13.84300000000000530, 1.648619521012166368E-15 ) ) ;
#35478=DIRECTION ( 'NONE',  ( 0.000000000000000000, 1.000000000000000000, 0.000000000000000000 ) ) ;
#35511=CIRCLE ( 'NONE', #4209, 14.09699999999999420 ) ;
#35518=CARTESIAN_POINT ( 'NONE',  ( 6.059261036834406866, 57.14999999999999858, -5.016499999999999737 ) ) ;
#35524=CARTESIAN_POINT ( 'NONE',  ( 20.83467972660109524, 65.95194780259438971, 1.904999999999986704 ) ) ;
#35525=EDGE_CURVE ( 'NONE', #11643, #19019, #3090, .T. ) ;
#35533=CARTESIAN_POINT ( 'NONE',  ( -18.35410564743290607, 77.35382415001784295, 5.016499999999999737 ) ) ;
#35548=CARTESIAN_POINT ( 'NONE',  ( 4.997525182441497016, 56.61525291752807476, 5.184946129310834984 ) ) ;
#35554=CARTESIAN_POINT ( 'NONE',  ( 12.21488373879588885, 56.36092316367926713, -5.016500000000000625 ) ) ;
#35558=ORIENTED_EDGE ( 'NONE', *, *, #19352, .T. ) ;
#35562=CARTESIAN_POINT ( 'NONE',  ( -5.583532163260057857, 78.91300747758680245, -5.082153855702578937 ) ) ;
#35577=DIRECTION ( 'NONE',  ( 1.000000000000000000, 0.000000000000000000, -1.224646799147353947E-16 ) ) ;
#35589=ORIENTED_EDGE ( 'NONE', *, *, #28433, .F. ) ;
#35590=ORIENTED_EDGE ( 'NONE', *, *, #25005, .F. ) ;
#35631=CARTESIAN_POINT ( 'NONE',  ( 5.305748947172213015, 53.58606249999999704, 5.247078976224250013 ) ) ;
#35640=EDGE_LOOP ( 'NONE', ( #6176, #13640, #23807, #29397 ) ) ;
#35646=( BOUNDED_CURVE ( )  B_SPLINE_CURVE ( 3, ( #39324, #20327, #33150, #23522 ),
 .UNSPECIFIED., .F., .T. ) 
 B_SPLINE_CURVE_WITH_KNOTS ( ( 4, 4 ),
 ( 3.141592653589793560, 4.712388980384689674 ),
 .UNSPECIFIED. ) 
 CURVE ( )  GEOMETRIC_REPRESENTATION_ITEM ( )  RATIONAL_B_SPLINE_CURVE ( ( 1.000000000000000000, 0.8047378541243650485, 0.8047378541243650485, 1.000000000000000000 ) ) 
 REPRESENTATION_ITEM ( '' )  );
#35660=DIRECTION ( 'NONE',  ( -0.000000000000000000, -0.000000000000000000, -1.000000000000000000 ) ) ;
#35663=FACE_OUTER_BOUND ( 'NONE', #27607, .T. ) ;
#35664=TOROIDAL_SURFACE ( 'NONE', #31577, 17.68910244842765778, 0.6350000000000000089 ) ;
#35671=CARTESIAN_POINT ( 'NONE',  ( 18.35410564743290607, 77.35382415001784295, 5.016499999999999737 ) ) ;
#35674=CARTESIAN_POINT ( 'NONE',  ( -5.871452009091403745, 88.73331249999998249, 5.016499999999999737 ) ) ;
#35687=FACE_OUTER_BOUND ( 'NONE', #41733, .T. ) ;
#35693=LINE ( 'NONE', #2695, #2554 ) ;
#35698=LINE ( 'NONE', #19277, #38167 ) ;
#35723=CARTESIAN_POINT ( 'NONE',  ( 5.177913976931214357, 57.14999999999996305, -5.372099999999997877 ) ) ;
#35727=EDGE_LOOP ( 'NONE', ( #23332, #37446, #13606, #25956 ) ) ;
#35743=CARTESIAN_POINT ( 'NONE',  ( -14.73199999999999754, 61.59499999999999886, -5.016499999999999737 ) ) ;
#35757=DIRECTION ( 'NONE',  ( -0.000000000000000000, -0.000000000000000000, -1.000000000000000000 ) ) ;
#35761=CARTESIAN_POINT ( 'NONE',  ( -5.450291846086723346, 56.51500000000001478, -4.451173312910844615 ) ) ;
#35785=( NAMED_UNIT ( * ) SI_UNIT ( $, .STERADIAN. ) SOLID_ANGLE_UNIT ( ) );
#35787=VECTOR ( 'NONE', #37939, 1000.000000000000000 ) ;
#35822=CONICAL_SURFACE ( 'NONE', #12002, 14.73199999999999577, 0.7853981633974488341 ) ;
#35843=ORIENTED_EDGE ( 'NONE', *, *, #26054, .F. ) ;
#35844=CARTESIAN_POINT ( 'NONE',  ( 5.177913976931209916, 65.30181249999998272, 5.372099999999993436 ) ) ;
#35847=CARTESIAN_POINT ( 'NONE',  ( -14.39766717389551864, 57.78499999999998948, 1.905000000000000471 ) ) ;
#35852=CARTESIAN_POINT ( 'NONE',  ( 5.901202670473767675, 78.88741954747038676, 5.016800487701043920 ) ) ;
#35853=ORIENTED_EDGE ( 'NONE', *, *, #5023, .F. ) ;
#35866=ORIENTED_EDGE ( 'NONE', *, *, #38882, .T. ) ;
#35871=CIRCLE ( 'NONE', #18174, 17.68910244842765778 ) ;
#35875=LINE ( 'NONE', #9453, #39639 ) ;
#35887=CARTESIAN_POINT ( 'NONE',  ( -5.871452009091383317, 53.58606250000000415, 5.016499999999999737 ) ) ;
#35905=DIRECTION ( 'NONE',  ( 1.000000000000000000, 0.000000000000000000, 0.000000000000000000 ) ) ;
#35908=CARTESIAN_POINT ( 'NONE',  ( -13.85159022459153988, 16.51000000000000156, 5.016499999999999737 ) ) ;
#35912=VERTEX_POINT ( 'NONE', #7956 ) ;
#35923=VERTEX_POINT ( 'NONE', #33947 ) ;
#35950=CARTESIAN_POINT ( 'NONE',  ( 7.213960532363565825, 86.35999999999998522, 1.904999999999995364 ) ) ;
#35971=DIRECTION ( 'NONE',  ( 5.463695987328526437E-16, 1.000000000000000000, 1.672774450599033775E-31 ) ) ;
#35972=LINE ( 'NONE', #25738, #16769 ) ;
#35974=DIRECTION ( 'NONE',  ( -0.000000000000000000, 1.000000000000000000, 0.000000000000000000 ) ) ;
#35991=DIRECTION ( 'NONE',  ( 0.000000000000000000, 1.000000000000000000, 0.000000000000000000 ) ) ;
#36023=EDGE_CURVE ( 'NONE', #20064, #4948, #4183, .T. ) ;
#36027=CARTESIAN_POINT ( 'NONE',  ( 10.28897677580358128, 57.14999999999999858, 5.016499999999999737 ) ) ;
#36032=DIRECTION ( 'NONE',  ( 0.000000000000000000, 0.000000000000000000, 1.000000000000000000 ) ) ;
#36043=CARTESIAN_POINT ( 'NONE',  ( -11.04921058900168873, 56.51499999999998636, -4.436160551868583823 ) ) ;
#36051=DIRECTION ( 'NONE',  ( -5.463695987328526437E-16, -1.000000000000000000, -1.672774450599033775E-31 ) ) ;
#36052=VECTOR ( 'NONE', #39787, 1000.000000000000000 ) ;
#36054=DIRECTION ( 'NONE',  ( -1.000000000000000000, -6.353134868986659519E-16, 0.000000000000000000 ) ) ;
#36071=VERTEX_POINT ( 'NONE', #54 ) ;
#36098=CARTESIAN_POINT ( 'NONE',  ( -18.35410564743290962, 77.35382415001784295, -5.392902600000144986 ) ) ;
#36114=DIRECTION ( 'NONE',  ( -1.000000000000000000, 0.000000000000000000, -5.975917486140574681E-16 ) ) ;
#36118=DIRECTION ( 'NONE',  ( -1.000000000000000000, 1.893378931774809890E-16, 0.000000000000000000 ) ) ;
#36123=CARTESIAN_POINT ( 'NONE',  ( -5.451267667241070720E-14, 85.80437499999999318, 0.000000000000000000 ) ) ;
#36141=EDGE_CURVE ( 'NONE', #24583, #25879, #12410, .T. ) ;
#36143=DIRECTION ( 'NONE',  ( -6.853480209240093652E-32, -1.000000000000000000, 3.905054717696927820E-31 ) ) ;
#36169=CARTESIAN_POINT ( 'NONE',  ( 6.059261036834406866, 56.51500000000000057, 4.381500000000000838 ) ) ;
#36174=ORIENTED_EDGE ( 'NONE', *, *, #37572, .T. ) ;
#36182=CARTESIAN_POINT ( 'NONE',  ( -18.35410564743290962, 77.35382415001784295, 5.392902600000138769 ) ) ;
#36189=CARTESIAN_POINT ( 'NONE',  ( -5.511339492779010030, 57.15000000000000568, -5.111277471990291588 ) ) ;
#36196=CARTESIAN_POINT ( 'NONE',  ( -6.059261036834082681, 78.87450423423038615, -5.016499999999999737 ) ) ;
#36197=ORIENTED_EDGE ( 'NONE', *, *, #40973, .F. ) ;
#36229=ADVANCED_FACE ( 'NONE', ( #33056, #10880 ), #13661, .F. ) ;
#36234=ORIENTED_EDGE ( 'NONE', *, *, #31090, .F. ) ;
#36237=CARTESIAN_POINT ( 'NONE',  ( 18.35410564743290607, 77.35382415001784295, 5.016499999999999737 ) ) ;
#36238=B_SPLINE_CURVE_WITH_KNOTS ( 'NONE', 3,
 ( #35533, #9128, #12730, #25719 ),
 .UNSPECIFIED., .F., .F.,
 ( 4, 4 ),
 ( 0.000000000000000000, 0.5643836377221552736 ),
 .UNSPECIFIED. ) ;
#36239=CYLINDRICAL_SURFACE ( 'NONE', #13650, 6.350000000000004974 ) ;
#36252=CARTESIAN_POINT ( 'NONE',  ( -10.63219908769152866, 56.50600268266023107, -5.016499999999338932 ) ) ;
#36264=ORIENTED_EDGE ( 'NONE', *, *, #16689, .F. ) ;
#36287=VERTEX_POINT ( 'NONE', #7704 ) ;
#36304=CIRCLE ( 'NONE', #10448, 6.350000000000004974 ) ;
#36332=CARTESIAN_POINT ( 'NONE',  ( -11.04921058900168873, 56.51499999999998636, 4.436160551868583823 ) ) ;
#36361=ADVANCED_FACE ( 'NONE', ( #4515 ), #37619, .T. ) ;
#36365=EDGE_LOOP ( 'NONE', ( #18959, #21214 ) ) ;
#36368=ORIENTED_EDGE ( 'NONE', *, *, #10027, .F. ) ;
#36377=EDGE_CURVE ( 'NONE', #6797, #32761, #3255, .T. ) ;
#36378=EDGE_LOOP ( 'NONE', ( #32476, #19726, #3750, #26713 ) ) ;
#36381=DIRECTION ( 'NONE',  ( 9.627370216492862708E-17, 1.000000000000000000, -0.000000000000000000 ) ) ;
#36382=CARTESIAN_POINT ( 'NONE',  ( -20.83467972660109524, 65.95194780259438971, 1.904999999999986704 ) ) ;
#36387=CARTESIAN_POINT ( 'NONE',  ( 5.638212235186404797, 57.14999999999997016, 5.060089761242341666 ) ) ;
#36391=ORIENTED_EDGE ( 'NONE', *, *, #40491, .F. ) ;
#36407=CARTESIAN_POINT ( 'NONE',  ( 13.85159022459153988, 59.63164443796365077, 5.016499999999999737 ) ) ;
#36412=ORIENTED_EDGE ( 'NONE', *, *, #38386, .T. ) ;
#36448=CARTESIAN_POINT ( 'NONE',  ( -6.059261036834475256, 57.15000000000000568, 5.016499999999999737 ) ) ;
#36449=LINE ( 'NONE', #9606, #35455 ) ;
#36453=CARTESIAN_POINT ( 'NONE',  ( 14.95453923199683111, 61.75387968257833649, -5.016499999999999737 ) ) ;
#36462=CARTESIAN_POINT ( 'NONE',  ( -10.45888906141536268, 56.51499999999998636, -4.393716635381741398 ) ) ;
#36472=ORIENTED_EDGE ( 'NONE', *, *, #38882, .F. ) ;
#36479=ORIENTED_EDGE ( 'NONE', *, *, #39925, .F. ) ;
#36491=AXIS2_PLACEMENT_3D ( 'NONE', #2248, #18614, #21373 ) ;
#36495=DIRECTION ( 'NONE',  ( 0.000000000000000000, 0.000000000000000000, 1.000000000000000000 ) ) ;
#36511=CARTESIAN_POINT ( 'NONE',  ( -9.094996104468901166, 78.64197151092922411, -1.904999999999999583 ) ) ;
#36521=CARTESIAN_POINT ( 'NONE',  ( -12.69999999999999574, 14.60500000000000398, 0.000000000000000000 ) ) ;
#36531=EDGE_CURVE ( 'NONE', #10259, #24258, #22258, .T. ) ;
#36559=ADVANCED_FACE ( 'NONE', ( #37289 ), #27498, .F. ) ;
#36564=FACE_OUTER_BOUND ( 'NONE', #19233, .T. ) ;
#36575=CARTESIAN_POINT ( 'NONE',  ( -6.608367952640316290, 78.82866613109548837, -3.480504251946396455 ) ) ;
#36602=LINE ( 'NONE', #24212, #23202 ) ;
#36604=EDGE_CURVE ( 'NONE', #17420, #19292, #21492, .T. ) ;
#36608=EDGE_CURVE ( 'NONE', #27525, #42131, #5558, .T. ) ;
#36628=CARTESIAN_POINT ( 'NONE',  ( -13.34597544948414694, 17.14500000000000313, -5.016499999999999737 ) ) ;
#36640=ORIENTED_EDGE ( 'NONE', *, *, #375, .T. ) ;
#36664=CARTESIAN_POINT ( 'NONE',  ( 11.48503488083560597, 55.92196062030126313, 5.016500000000108095 ) ) ;
#36667=EDGE_LOOP ( 'NONE', ( #35590, #19904, #28281, #16403 ) ) ;
#36687=DIRECTION ( 'NONE',  ( 1.000000000000000000, -9.627370216492862708E-17, 0.000000000000000000 ) ) ;
#36701=LINE ( 'NONE', #40740, #40185 ) ;
#36710=VECTOR ( 'NONE', #37956, 1000.000000000000114 ) ;
#36720=PLANE ( 'NONE',  #15051 ) ;
#36722=DIRECTION ( 'NONE',  ( -0.1469470846586743706, -9.335746474409589170E-17, 0.9891443546370348727 ) ) ;
#36740=EDGE_LOOP ( 'NONE', ( #9899, #12783, #19554, #19805 ) ) ;
#36744=ADVANCED_FACE ( 'NONE', ( #15742 ), #42026, .T. ) ;
#36764=DIRECTION ( 'NONE',  ( -1.000000000000000000, -9.299908063537918137E-16, 0.000000000000000000 ) ) ;
#36768=EDGE_CURVE ( 'NONE', #26876, #27491, #32502, .T. ) ;
#36770=CARTESIAN_POINT ( 'NONE',  ( 5.871452009091314039, 57.14999999999998437, 5.016499999999999737 ) ) ;
#36776=EDGE_CURVE ( 'NONE', #40888, #17420, #38969, .T. ) ;
#36780=ORIENTED_EDGE ( 'NONE', *, *, #31099, .T. ) ;
#36792=CARTESIAN_POINT ( 'NONE',  ( 13.77279150232676130, 16.85108474679722690, 5.016499999999997961 ) ) ;
#36807=VECTOR ( 'NONE', #25174, 1000.000000000000114 ) ;
#36852=EDGE_CURVE ( 'NONE', #38115, #20064, #28393, .T. ) ;
#36872=AXIS2_PLACEMENT_3D ( 'NONE', #3656, #676, #30251 ) ;
#36878=FACE_BOUND ( 'NONE', #13157, .T. ) ;
#36885=CARTESIAN_POINT ( 'NONE',  ( -5.421568387540222744, 78.92574702321228131, 5.165409981420495455 ) ) ;
#36886=DIRECTION ( 'NONE',  ( 0.000000000000000000, 0.000000000000000000, 1.000000000000000000 ) ) ;
#36910=CARTESIAN_POINT ( 'NONE',  ( 20.83467972660109169, 65.95194780259438971, 5.016499999999999737 ) ) ;
#36915=CARTESIAN_POINT ( 'NONE',  ( 11.58677707360115861, 55.41127257906217807, -4.474811398756807002 ) ) ;
#36929=DIRECTION ( 'NONE',  ( -1.000000000000000000, -6.353134868986659519E-16, 0.000000000000000000 ) ) ;
#36933=CARTESIAN_POINT ( 'NONE',  ( -5.353961913965729735, 57.14999999999999858, 5.213928161019513396 ) ) ;
#36934=CARTESIAN_POINT ( 'NONE',  ( 18.32410244842765934, 17.14499999999999602, 2.244055341071511024E-15 ) ) ;
#36938=ORIENTED_EDGE ( 'NONE', *, *, #36776, .T. ) ;
#36941=ORIENTED_EDGE ( 'NONE', *, *, #36852, .F. ) ;
#36942=LINE ( 'NONE', #24345, #38971 ) ;
#36969=DIRECTION ( 'NONE',  ( 9.627370216492862708E-17, 1.000000000000000000, -0.000000000000000000 ) ) ;
#36974=DIRECTION ( 'NONE',  ( -1.000000000000000000, 0.000000000000000000, 0.000000000000000000 ) ) ;
#36983=AXIS2_PLACEMENT_3D ( 'NONE', #305, #13275, #36495 ) ;
#36994=CARTESIAN_POINT ( 'NONE',  ( -6.758480964575440453, 78.81581826900305998, -3.179117336685193695 ) ) ;
#37001=CARTESIAN_POINT ( 'NONE',  ( -7.213960532363665301, 83.56599999999998829, 1.904999999999995364 ) ) ;
#37012=ORIENTED_EDGE ( 'NONE', *, *, #931, .T. ) ;
#37024=CARTESIAN_POINT ( 'NONE',  ( -4.792324638262678960, 56.51998046905272588, 4.972049999962470324 ) ) ;
#37027=EDGE_CURVE ( 'NONE', #38485, #32125, #39277, .T. ) ;
#37029=LINE ( 'NONE', #8249, #1573 ) ;
#37051=CARTESIAN_POINT ( 'NONE',  ( -10.28897677580358305, 57.14999999999998437, -5.016499999999999737 ) ) ;
#37055=CARTESIAN_POINT ( 'NONE',  ( 5.241362157049057835, 53.58606249999999704, -5.310945289804168468 ) ) ;
#37068=ORIENTED_EDGE ( 'NONE', *, *, #4319, .F. ) ;
#37100=CARTESIAN_POINT ( 'NONE',  ( 10.28897677580358128, 57.14999999999999858, 5.016499999999999737 ) ) ;
#37110=FACE_OUTER_BOUND ( 'NONE', #19260, .T. ) ;
#37116=ADVANCED_FACE ( 'NONE', ( #26235 ), #23161, .T. ) ;
#37119=CARTESIAN_POINT ( 'NONE',  ( 10.96186877710200491, 56.39406130473815892, -5.016499999999892268 ) ) ;
#37128=CARTESIAN_POINT ( 'NONE',  ( -11.11710224467008601, 56.30409367656574915, 5.016499999999452619 ) ) ;
#37132=CARTESIAN_POINT ( 'NONE',  ( 11.66725022231030984, 16.51000000000000156, 5.016499999999999737 ) ) ;
#37144=EDGE_LOOP ( 'NONE', ( #24133, #22559, #21465, #4703 ) ) ;
#37150=LINE ( 'NONE', #17542, #6742 ) ;
#37173=DIRECTION ( 'NONE',  ( 1.000000000000000000, 0.000000000000000000, 0.000000000000000000 ) ) ;
#37178=CARTESIAN_POINT ( 'NONE',  ( 1.589478822742971486E-15, 16.51000000000000156, 0.000000000000000000 ) ) ;
#37197=ORIENTED_EDGE ( 'NONE', *, *, #33925, .F. ) ;
#37201=EDGE_LOOP ( 'NONE', ( #41099, #3594, #13967, #41117 ) ) ;
#37203=ORIENTED_EDGE ( 'NONE', *, *, #406, .T. ) ;
#37226=CARTESIAN_POINT ( 'NONE',  ( 1.650612623617701257E-15, 17.14499999999999957, 0.000000000000000000 ) ) ;
#37236=AXIS2_PLACEMENT_3D ( 'NONE', #19420, #36051, #19622 ) ;
#37248=DIRECTION ( 'NONE',  ( -1.000000000000000000, -1.092739197465705287E-15, 0.000000000000000000 ) ) ;
#37250=CARTESIAN_POINT ( 'NONE',  ( -12.21488373879589240, 55.24499999999999034, -5.016499999999999737 ) ) ;
#37254=CARTESIAN_POINT ( 'NONE',  ( 5.664977208693820820, 53.58606249999999704, -5.033228321271210781 ) ) ;
#37275=EDGE_CURVE ( 'NONE', #27765, #5344, #29331, .T. ) ;
#37289=FACE_OUTER_BOUND ( 'NONE', #40407, .T. ) ;
#37312=DIRECTION ( 'NONE',  ( -6.353134868986659519E-16, 1.000000000000000000, -0.000000000000000000 ) ) ;
#37317=CARTESIAN_POINT ( 'NONE',  ( 11.58677707360137710, 55.24500000000000455, 4.474811398758258285 ) ) ;
#37325=VECTOR ( 'NONE', #14266, 1000.000000000000000 ) ;
#37334=CARTESIAN_POINT ( 'NONE',  ( -11.82906070755491612, 56.41571150956222880, 5.016499999999999737 ) ) ;
#37341=CARTESIAN_POINT ( 'NONE',  ( -5.177913976931285411, 57.14999999999999858, -5.372100000000001430 ) ) ;
#37347=EDGE_LOOP ( 'NONE', ( #38412, #6159, #19986, #13484 ) ) ;
#37367=EDGE_CURVE ( 'NONE', #42131, #11710, #24303, .T. ) ;
#37369=ORIENTED_EDGE ( 'NONE', *, *, #7992, .T. ) ;
#37398=CARTESIAN_POINT ( 'NONE',  ( 1.204770341778093456E-15, 12.51401280605345967, 0.000000000000000000 ) ) ;
#37404=AXIS2_PLACEMENT_3D ( 'NONE', #18761, #36969, #5384 ) ;
#37417=VERTEX_POINT ( 'NONE', #7918 ) ;
#37421=EDGE_LOOP ( 'NONE', ( #5260, #31371, #10895, #22601 ) ) ;
#37424=DIRECTION ( 'NONE',  ( -1.000000000000000000, 0.000000000000000000, 0.000000000000000000 ) ) ;
#37428=LINE ( 'NONE', #5709, #28767 ) ;
#37430=CARTESIAN_POINT ( 'NONE',  ( 5.813441077436474202, 56.51500000000003610, -4.384678760708148992 ) ) ;
#37437=VERTEX_POINT ( 'NONE', #37100 ) ;
#37440=DIRECTION ( 'NONE',  ( -0.000000000000000000, -0.000000000000000000, -1.000000000000000000 ) ) ;
#37446=ORIENTED_EDGE ( 'NONE', *, *, #38355, .T. ) ;
#37455=CARTESIAN_POINT ( 'NONE',  ( 5.664977208693820820, 65.30181249999998272, -5.033228321271210781 ) ) ;
#37462=B_SPLINE_CURVE_WITH_KNOTS ( 'NONE', 3,
 ( #9068, #19052, #22653, #19680, #41876, #29066 ),
 .UNSPECIFIED., .F., .F.,
 ( 4, 2, 4 ),
 ( 8.339423840660491790E-05, 0.0004508778365104737095, 0.0008183614346143424333 ),
 .UNSPECIFIED. ) ;
#37476=FACE_OUTER_BOUND ( 'NONE', #32635, .T. ) ;
#37483=CARTESIAN_POINT ( 'NONE',  ( 11.25890006629630591, 56.90956307411710924, 5.016499999999999737 ) ) ;
#37487=ORIENTED_EDGE ( 'NONE', *, *, #18338, .F. ) ;
#37508=AXIS2_PLACEMENT_3D ( 'NONE', #7930, #34752, #8769 ) ;
#37516=DIRECTION ( 'NONE',  ( 0.000000000000000000, -0.000000000000000000, -1.000000000000000000 ) ) ;
#37519=VECTOR ( 'NONE', #2719, 1000.000000000000000 ) ;
#37527=CARTESIAN_POINT ( 'NONE',  ( 11.25890006629607143, 56.90956307411702397, -5.016500000000000625 ) ) ;
#37533=AXIS2_PLACEMENT_3D ( 'NONE', #15102, #28534, #11493 ) ;
#37548=DIRECTION ( 'NONE',  ( 9.627370216492862708E-17, 1.000000000000000000, -0.000000000000000000 ) ) ;
#37554=ORIENTED_EDGE ( 'NONE', *, *, #23278, .F. ) ;
#37572=EDGE_CURVE ( 'NONE', #4432, #31634, #31900, .T. ) ;
#37587=EDGE_CURVE ( 'NONE', #16646, #6407, #28957, .T. ) ;
#37589=ORIENTED_EDGE ( 'NONE', *, *, #11735, .T. ) ;
#37593=EDGE_CURVE ( 'NONE', #5725, #22720, #32399, .T. ) ;
#37617=VERTEX_POINT ( 'NONE', #2794 ) ;
#37619=( BOUNDED_SURFACE ( )  B_SPLINE_SURFACE ( 3, 2, ( 
 ( #26441, #29643, #10248 ),
 ( #36462, #26865, #20243 ),
 ( #39873, #36252, #4098 ),
 ( #7074, #20037, #8317 ),
 ( #14485, #11300, #40706 ),
 ( #5350, #1529, #40299 ),
 ( #18514, #31306, #18100 ),
 ( #31103, #18304, #34107 ),
 ( #8532, #34524, #31520 ),
 ( #27904, #1942, #14693 ) ),
 .UNSPECIFIED., .F., .F., .F. ) 
 B_SPLINE_SURFACE_WITH_KNOTS ( ( 4, 2, 2, 2, 4 ),
 ( 3, 3 ),
 ( 4.712388980384689674, 5.105088062083413369, 5.497787143782137065, 5.890486225480861648, 6.283185307179585344 ),
 ( 0.000000000000000000, 1.000000000000000000 ),
 .UNSPECIFIED. ) 
 GEOMETRIC_REPRESENTATION_ITEM ( )  RATIONAL_B_SPLINE_SURFACE ( (
 ( 1.000000000000000000, 0.7071067811865475727, 1.000000000000000000),
 ( 1.000000000000000000, 0.7139102541738931995, 1.000000000000000000),
 ( 1.000000000000000000, 0.7206031636702244780, 1.000000000000000000),
 ( 1.000000000000000000, 0.7328301610703541469, 1.000000000000000000),
 ( 1.000000000000000000, 0.7383589052088842530, 1.000000000000000000),
 ( 1.000000000000000000, 0.7475127447244133139, 1.000000000000000000),
 ( 1.000000000000000000, 0.7511365686958336729, 1.000000000000000000),
 ( 1.000000000000000000, 0.7560206254138944759, 1.000000000000000000),
 ( 1.000000000000000000, 0.7572851909593535380, 1.000000000000000000),
 ( 1.000000000000000000, 0.7572803591334833495, 1.000000000000000000) ) ) 
 REPRESENTATION_ITEM ( '' )  SURFACE ( )  );
#37634=CIRCLE ( 'NONE', #11082, 6.349999999999999645 ) ;
#37645=CARTESIAN_POINT ( 'NONE',  ( 10.92199999999999704, 12.96416000000000146, 0.000000000000000000 ) ) ;
#37646=B_SPLINE_CURVE_WITH_KNOTS ( 'NONE', 3,
 ( #38948, #19749, #35548, #19334, #10176, #31928 ),
 .UNSPECIFIED., .F., .F.,
 ( 4, 2, 4 ),
 ( 0.07978617534938510503, 0.5398930876746925733, 1.000000000000000000 ),
 .UNSPECIFIED. ) ;
#37648=FACE_OUTER_BOUND ( 'NONE', #11709, .T. ) ;
#37650=CARTESIAN_POINT ( 'NONE',  ( 5.177913976931208140, 64.41499993257285439, 5.372100000000000541 ) ) ;
#37663=ORIENTED_EDGE ( 'NONE', *, *, #3477, .T. ) ;
#37685=VERTEX_POINT ( 'NONE', #39616 ) ;
#37698=CARTESIAN_POINT ( 'NONE',  ( -5.256666790930538014, 56.51500000000019952, -5.296388420399792629 ) ) ;
#37700=CARTESIAN_POINT ( 'NONE',  ( 11.08653569745430190, 56.26057688450594441, 4.438844214435382796 ) ) ;
#37703=ORIENTED_EDGE ( 'NONE', *, *, #15180, .T. ) ;
#37704=EDGE_LOOP ( 'NONE', ( #9384, #40632, #23735, #23199, #8754, #34051, #31327, #3733 ) ) ;
#37709=CARTESIAN_POINT ( 'NONE',  ( -17.14499999999999957, 71.11999999999999034, 1.904999999999989146 ) ) ;
#37717=CARTESIAN_POINT ( 'NONE',  ( -14.73199999999999932, 12.96416000000000146, 0.000000000000000000 ) ) ;
#37728=ORIENTED_EDGE ( 'NONE', *, *, #16581, .T. ) ;
#37737=CYLINDRICAL_SURFACE ( 'NONE', #32451, 6.350000000000004974 ) ;
#37738=B_SPLINE_CURVE_WITH_KNOTS ( 'NONE', 3,
 ( #23083, #10535, #13734, #4382 ),
 .UNSPECIFIED., .F., .F.,
 ( 4, 4 ),
 ( 0.000000000000000000, 0.9716004430332778607 ),
 .UNSPECIFIED. ) ;
#37755=FACE_OUTER_BOUND ( 'NONE', #15962, .T. ) ;
#37784=ORIENTED_EDGE ( 'NONE', *, *, #29434, .T. ) ;
#37791=CARTESIAN_POINT ( 'NONE',  ( -14.60500000000000043, 71.11999999999999034, 1.904999999999990701 ) ) ;
#37798=CARTESIAN_POINT ( 'NONE',  ( 15.50061618130081165, 62.14374591690594940, -1.904999999999999583 ) ) ;
#37808=CARTESIAN_POINT ( 'NONE',  ( 16.04309792416813707, 12.96416000000000146, 5.016499999999999737 ) ) ;
#37825=CARTESIAN_POINT ( 'NONE',  ( -19.68500000000000227, 71.11999999999999034, -1.904999999999999583 ) ) ;
#37833=EDGE_CURVE ( 'NONE', #33026, #10948, #39241, .T. ) ;
#37839=DIRECTION ( 'NONE',  ( -1.000000000000000000, 1.177520686924251719E-16, 0.000000000000000000 ) ) ;
#37843=VECTOR ( 'NONE', #5581, 1000.000000000000114 ) ;
#37855=CARTESIAN_POINT ( 'NONE',  ( 4.965996940879040977, 56.51499999999996504, -4.710730864944427942 ) ) ;
#37867=LINE ( 'NONE', #8486, #24598 ) ;
#37870=CARTESIAN_POINT ( 'NONE',  ( -6.756648348127426651, 78.81597664337222398, 3.183520453979958642 ) ) ;
#37902=CARTESIAN_POINT ( 'NONE',  ( 17.14499999999999957, 71.11999999999999034, 1.904999999999989146 ) ) ;
#37909=FACE_OUTER_BOUND ( 'NONE', #32167, .T. ) ;
#37911=ORIENTED_EDGE ( 'NONE', *, *, #38386, .F. ) ;
#37917=DIRECTION ( 'NONE',  ( -0.1715592850456333085, 0.1224830539174543292, -0.9775302108976914317 ) ) ;
#37931=ORIENTED_EDGE ( 'NONE', *, *, #33723, .T. ) ;
#37939=DIRECTION ( 'NONE',  ( -0.000000000000000000, -0.000000000000000000, -1.000000000000000000 ) ) ;
#37942=( LENGTH_UNIT ( ) NAMED_UNIT ( * ) SI_UNIT ( .MILLI., .METRE. ) );
#37954=VERTEX_POINT ( 'NONE', #11050 ) ;
#37956=DIRECTION ( 'NONE',  ( 0.1469470846586743706, -1.414713986243376972E-17, -0.9891443546370348727 ) ) ;
#37957=FACE_OUTER_BOUND ( 'NONE', #28740, .T. ) ;
#37962=DIRECTION ( 'NONE',  ( -0.000000000000000000, -0.000000000000000000, -1.000000000000000000 ) ) ;
#37975=FACE_OUTER_BOUND ( 'NONE', #3994, .T. ) ;
#37978=B_SPLINE_CURVE_WITH_KNOTS ( 'NONE', 3,
 ( #27888, #34507, #28312, #41320, #12124, #25114 ),
 .UNSPECIFIED., .F., .F.,
 ( 4, 2, 4 ),
 ( 0.000000000000000000, 0.0003611586812565004178, 0.0007223173625130008355 ),
 .UNSPECIFIED. ) ;
#37981=ORIENTED_EDGE ( 'NONE', *, *, #27362, .T. ) ;
#37993=CARTESIAN_POINT ( 'NONE',  ( -23.49500000000000455, 71.11999999999999034, -5.016499999999999737 ) ) ;
#38005=CIRCLE ( 'NONE', #3326, 6.350000000000004974 ) ;
#38020=CARTESIAN_POINT ( 'NONE',  ( -5.241362157049148429, 88.73331249999999670, -5.310945289804168468 ) ) ;
#38027=LINE ( 'NONE', #8210, #12178 ) ;
#38028=ORIENTED_EDGE ( 'NONE', *, *, #33827, .F. ) ;
#38036=DIRECTION ( 'NONE',  ( -1.000000000000000000, 0.000000000000000000, 0.000000000000000000 ) ) ;
#38059=EDGE_CURVE ( 'NONE', #18509, #35273, #4683, .T. ) ;
#38063=CARTESIAN_POINT ( 'NONE',  ( 1.406077420118782567E-15, 14.60500000000000220, 0.000000000000000000 ) ) ;
#38069=EDGE_CURVE ( 'NONE', #29870, #22529, #14442, .T. ) ;
#38070=FACE_OUTER_BOUND ( 'NONE', #30628, .T. ) ;
#38073=EDGE_CURVE ( 'NONE', #26298, #25879, #4543, .T. ) ;
#38076=CARTESIAN_POINT ( 'NONE',  ( -5.450166374333774044, 56.51499999999997215, 4.451212169035321686 ) ) ;
#38082=CARTESIAN_POINT ( 'NONE',  ( -13.17422243436020857, 17.14500000000000668, 5.016499999999999737 ) ) ;
#38087=ORIENTED_EDGE ( 'NONE', *, *, #22936, .T. ) ;
#38090=CARTESIAN_POINT ( 'NONE',  ( -3.671158984043940170E-14, 57.78499999999999659, 0.000000000000000000 ) ) ;
#38091=CARTESIAN_POINT ( 'NONE',  ( 7.213960532363571154, 78.77618639008812806, -1.904999999999999583 ) ) ;
#38112=ADVANCED_FACE ( 'NONE', ( #22084 ), #20824, .F. ) ;
#38114=AXIS2_PLACEMENT_3D ( 'NONE', #22573, #16621, #13228 ) ;
#38115=VERTEX_POINT ( 'NONE', #38720 ) ;
#38121=CARTESIAN_POINT ( 'NONE',  ( -11.97180806971945977, 56.20439414706015668, 5.016499999999999737 ) ) ;
#38145=CARTESIAN_POINT ( 'NONE',  ( -5.249547376985638891, 56.51499999999994373, 4.563748390655216980 ) ) ;
#38167=VECTOR ( 'NONE', #6723, 1000.000000000000000 ) ;
#38175=CARTESIAN_POINT ( 'NONE',  ( -10.92199999999999704, 12.96416000000000146, 0.000000000000000000 ) ) ;
#38199=ORIENTED_EDGE ( 'NONE', *, *, #18565, .F. ) ;
#38222=CIRCLE ( 'NONE', #26651, 6.985000000000000320 ) ;
#38239=CARTESIAN_POINT ( 'NONE',  ( -5.177913976931305839, 88.73331249999999670, -5.372100000000000541 ) ) ;
#38242=VERTEX_POINT ( 'NONE', #22498 ) ;
#38246=ORIENTED_EDGE ( 'NONE', *, *, #1749, .F. ) ;
#38255=CARTESIAN_POINT ( 'NONE',  ( 1.248107678658480997E-15, 12.96416000000000146, 0.000000000000000000 ) ) ;
#38273=DIRECTION ( 'NONE',  ( 1.000000000000000000, -1.288607544181256449E-16, 0.000000000000000000 ) ) ;
#38284=CARTESIAN_POINT ( 'NONE',  ( 5.941750549330224729, 56.51500000000122270, -5.016499812856827667 ) ) ;
#38288=CARTESIAN_POINT ( 'NONE',  ( -5.223971174379743232, 56.51499999999997215, 4.542495777410084479 ) ) ;
#38307=CARTESIAN_POINT ( 'NONE',  ( 5.322370863981891631, 57.14999999999997726, 5.239063870260719291 ) ) ;
#38343=DIRECTION ( 'NONE',  ( -0.8138664877804109299, -0.5810519254489895369, 0.000000000000000000 ) ) ;
#38351=LINE ( 'NONE', #29160, #5409 ) ;
#38352=LINE ( 'NONE', #24708, #24631 ) ;
#38355=EDGE_CURVE ( 'NONE', #3641, #19292, #3054, .T. ) ;
#38361=VERTEX_POINT ( 'NONE', #25085 ) ;
#38368=ORIENTED_EDGE ( 'NONE', *, *, #9517, .T. ) ;
#38372=( NAMED_UNIT ( * ) SI_UNIT ( $, .STERADIAN. ) SOLID_ANGLE_UNIT ( ) );
#38386=EDGE_CURVE ( 'NONE', #5419, #22830, #19317, .T. ) ;
#38389=CARTESIAN_POINT ( 'NONE',  ( -13.34597544948414161, 17.14500000000000313, 5.016499999999998849 ) ) ;
#38392=PLANE ( 'NONE',  #40998 ) ;
#38412=ORIENTED_EDGE ( 'NONE', *, *, #830, .F. ) ;
#38413=CARTESIAN_POINT ( 'NONE',  ( 6.059261036834384662, 77.01756249999996840, 5.016499999999999737 ) ) ;
#38426=DIRECTION ( 'NONE',  ( -1.000000000000000000, -9.933992704233682996E-16, 0.000000000000000000 ) ) ;
#38431=ORIENTED_EDGE ( 'NONE', *, *, #14841, .T. ) ;
#38436=DIRECTION ( 'NONE',  ( -1.000000000000000000, 0.000000000000000000, 0.000000000000000000 ) ) ;
#38448=DIRECTION ( 'NONE',  ( 0.1469470846586743706, 0.000000000000000000, -0.9891443546370348727 ) ) ;
#38449=CARTESIAN_POINT ( 'NONE',  ( -5.664977208693910526, 77.01756249999996840, -5.033228321271210781 ) ) ;
#38464=CARTESIAN_POINT ( 'NONE',  ( 7.213960532367366341, 78.77618639008778700, 1.904999999999999583 ) ) ;
#38467=FACE_OUTER_BOUND ( 'NONE', #17817, .T. ) ;
#38469=VECTOR ( 'NONE', #41294, 1000.000000000000000 ) ;
#38482=DIRECTION ( 'NONE',  ( -1.000000000000000000, 0.000000000000000000, -0.000000000000000000 ) ) ;
#38485=VERTEX_POINT ( 'NONE', #18037 ) ;
#38495=CARTESIAN_POINT ( 'NONE',  ( -2.032601633563780229E-14, 30.83083951148100255, -1.904999999999999805 ) ) ;
#38505=ORIENTED_EDGE ( 'NONE', *, *, #18547, .T. ) ;
#38521=AXIS2_PLACEMENT_3D ( 'NONE', #26057, #32255, #25643 ) ;
#38528=EDGE_CURVE ( 'NONE', #18529, #15597, #17621, .T. ) ;
#38531=CARTESIAN_POINT ( 'NONE',  ( 14.50851225146812595, 78.09971119798316863, 1.904999999999988258 ) ) ;
#38560=DIRECTION ( 'NONE',  ( -0.1728608224830406603, 0.000000000000000000, -0.9849462604886047856 ) ) ;
#38619=EDGE_CURVE ( 'NONE', #27003, #15597, #31282, .T. ) ;
#38620=VERTEX_POINT ( 'NONE', #19875 ) ;
#38628=ORIENTED_EDGE ( 'NONE', *, *, #19707, .F. ) ;
#38637=AXIS2_PLACEMENT_3D ( 'NONE', #34380, #2012, #31385 ) ;
#38644=DIRECTION ( 'NONE',  ( 1.000000000000000000, -9.466894658874049451E-17, 0.000000000000000000 ) ) ;
#38650=CARTESIAN_POINT ( 'NONE',  ( -18.35410564743290607, 77.35382415001784295, 5.016499999999999737 ) ) ;
#38651=EDGE_CURVE ( 'NONE', #31590, #19292, #23058, .T. ) ;
#38659=DIRECTION ( 'NONE',  ( 1.000000000000000000, -9.466894658874049451E-17, 0.000000000000000000 ) ) ;
#38662=ORIENTED_EDGE ( 'NONE', *, *, #23309, .T. ) ;
#38671=CARTESIAN_POINT ( 'NONE',  ( 6.059261036833980540, 78.87450423423040036, -5.016499999999999737 ) ) ;
#38682=ORIENTED_EDGE ( 'NONE', *, *, #38528, .F. ) ;
#38697=CARTESIAN_POINT ( 'NONE',  ( -12.21488373879589240, 55.24499999999999034, -5.016499999999999737 ) ) ;
#38714=ADVANCED_FACE ( 'NONE', ( #7761 ), #14330, .F. ) ;
#38715=ORIENTED_EDGE ( 'NONE', *, *, #36768, .T. ) ;
#38719=DIRECTION ( 'NONE',  ( -1.000000000000000000, 1.288607544181256696E-16, 0.000000000000000000 ) ) ;
#38720=CARTESIAN_POINT ( 'NONE',  ( -10.28897677580358305, 56.51499999999998636, 4.381500000000000838 ) ) ;
#38731=ORIENTED_EDGE ( 'NONE', *, *, #29800, .T. ) ;
#38743=AXIS2_PLACEMENT_3D ( 'NONE', #29729, #3557, #16516 ) ;
#38745=CIRCLE ( 'NONE', #2711, 2.540000000000000480 ) ;
#38748=DIRECTION ( 'NONE',  ( -9.627370216492862708E-17, -1.000000000000000000, 0.000000000000000000 ) ) ;
#38755=EDGE_LOOP ( 'NONE', ( #6116, #4855, #9545, #15056, #6920, #34446 ) ) ;
#38763=CARTESIAN_POINT ( 'NONE',  ( -6.059261036834476144, 56.51499999999998636, 4.547742611252458822 ) ) ;
#38767=CYLINDRICAL_SURFACE ( 'NONE', #10567, 1.270000000000000240 ) ;
#38781=CARTESIAN_POINT ( 'NONE',  ( -20.83467972660109169, 65.95194780259438971, 5.016499999999999737 ) ) ;
#38794=CARTESIAN_POINT ( 'NONE',  ( 11.58677707360137532, 55.98894877578617724, -4.474811398758259173 ) ) ;
#38802=CARTESIAN_POINT ( 'NONE',  ( -5.177913976931291629, 64.41499993257284018, -5.372099999999999653 ) ) ;
#38812=CARTESIAN_POINT ( 'NONE',  ( -10.28897677580358305, 56.51499999999998636, -4.381499999999999950 ) ) ;
#38821=CARTESIAN_POINT ( 'NONE',  ( 5.871452009091314039, 53.58606249999999704, 5.016499999999999737 ) ) ;
#38840=EDGE_LOOP ( 'NONE', ( #5235, #35033, #4484, #41408, #11813, #31832, #5330, #33264, #8123, #24777, #25975, #18695 ) ) ;
#38846=EDGE_CURVE ( 'NONE', #27765, #19376, #33875, .T. ) ;
#38861=DIRECTION ( 'NONE',  ( 1.000000000000000000, 6.353134868986659519E-16, 0.000000000000000000 ) ) ;
#38862=CARTESIAN_POINT ( 'NONE',  ( -5.241362157049125337, 65.30181249999996851, 5.310945289804168468 ) ) ;
#38875=DIRECTION ( 'NONE',  ( 1.000000000000000000, -1.288607544181256449E-16, 0.000000000000000000 ) ) ;
#38882=EDGE_CURVE ( 'NONE', #29870, #4305, #8541, .T. ) ;
#38883=LINE ( 'NONE', #29288, #3716 ) ;
#38900=CIRCLE ( 'NONE', #33465, 0.5556250000000014788 ) ;
#38901=FACE_OUTER_BOUND ( 'NONE', #38755, .T. ) ;
#38905=ADVANCED_FACE ( 'NONE', ( #3198 ), #38767, .F. ) ;
#38912=PLANE ( 'NONE',  #21264 ) ;
#38916=UNCERTAINTY_MEASURE_WITH_UNIT (LENGTH_MEASURE( 1.000000000000000082E-05 ), #19777, 'distance_accuracy_value', 'NONE');
#38926=EDGE_LOOP ( 'NONE', ( #25021, #23362, #34918, #21386 ) ) ;
#38935=CARTESIAN_POINT ( 'NONE',  ( 5.256666790930580646, 56.51499999999976609, 5.296388420400072405 ) ) ;
#38940=EDGE_CURVE ( 'NONE', #33497, #27131, #18947, .T. ) ;
#38948=CARTESIAN_POINT ( 'NONE',  ( 4.792324638247207780, 56.51998046905276141, 4.972049999977001811 ) ) ;
#38952=MANIFOLD_SOLID_BREP ( 'Stock-MAS-162-1', #33294 ) ;
#38953=AXIS2_PLACEMENT_3D ( 'NONE', #35446, #35241, #15416 ) ;
#38955=CARTESIAN_POINT ( 'NONE',  ( -5.860279866549801042, 57.14999999999999147, -5.019549989156839587 ) ) ;
#38956=DIRECTION ( 'NONE',  ( -6.353134868986659519E-16, 1.000000000000000000, -0.000000000000000000 ) ) ;
#38964=ORIENTED_EDGE ( 'NONE', *, *, #35338, .T. ) ;
#38969=LINE ( 'NONE', #15323, #6657 ) ;
#38971=VECTOR ( 'NONE', #14546, 1000.000000000000000 ) ;
#38995=( LENGTH_UNIT ( ) NAMED_UNIT ( * ) SI_UNIT ( .MILLI., .METRE. ) );
#39015=DIRECTION ( 'NONE',  ( -0.000000000000000000, -1.000000000000000000, -0.000000000000000000 ) ) ;
#39022=LINE ( 'NONE', #10039, #16206 ) ;
#39032=CARTESIAN_POINT ( 'NONE',  ( 5.241362157049057835, 53.58606249999999704, 5.310945289804168468 ) ) ;
#39041=ORIENTED_EDGE ( 'NONE', *, *, #20706, .F. ) ;
#39051=ORIENTED_EDGE ( 'NONE', *, *, #23543, .T. ) ;
#39065=AXIS2_PLACEMENT_3D ( 'NONE', #35272, #19687, #36118 ) ;
#39071=DIRECTION ( 'NONE',  ( -0.000000000000000000, -0.000000000000000000, -1.000000000000000000 ) ) ;
#39075=CARTESIAN_POINT ( 'NONE',  ( -5.664977208693910526, 88.73331249999998249, 5.033228321271210781 ) ) ;
#39097=ORIENTED_EDGE ( 'NONE', *, *, #36141, .F. ) ;
#39119=CARTESIAN_POINT ( 'NONE',  ( -7.213960532363670630, 78.77618639008812806, 1.904999999999999583 ) ) ;
#39123=EDGE_CURVE ( 'NONE', #21058, #31705, #39992, .T. ) ;
#39157=VECTOR ( 'NONE', #29116, 1000.000000000000000 ) ;
#39176=EDGE_CURVE ( 'NONE', #40534, #36287, #23151, .T. ) ;
#39186=VECTOR ( 'NONE', #34399, 1000.000000000000114 ) ;
#39200=ORIENTED_EDGE ( 'NONE', *, *, #33725, .T. ) ;
#39209=DIRECTION ( 'NONE',  ( 1.000000000000000000, 6.353134868986659519E-16, -0.000000000000000000 ) ) ;
#39215=DIRECTION ( 'NONE',  ( 0.000000000000000000, 1.000000000000000000, -0.000000000000000000 ) ) ;
#39238=DIRECTION ( 'NONE',  ( -0.000000000000000000, -1.000000000000000000, -0.000000000000000000 ) ) ;
#39240=CARTESIAN_POINT ( 'NONE',  ( 5.965356522962860453, 65.30181249999998272, 5.016499999999999737 ) ) ;
#39241=( BOUNDED_CURVE ( )  B_SPLINE_CURVE ( 3, ( #37051, #8491, #18472, #37250 ),
 .UNSPECIFIED., .F., .T. ) 
 B_SPLINE_CURVE_WITH_KNOTS ( ( 4, 4 ),
 ( 4.712388980384689674, 6.283185307179585344 ),
 .UNSPECIFIED. ) 
 CURVE ( )  GEOMETRIC_REPRESENTATION_ITEM ( )  RATIONAL_B_SPLINE_CURVE ( ( 1.000000000000000000, 0.8047378541243649375, 0.8047378541243649375, 1.000000000000000000 ) ) 
 REPRESENTATION_ITEM ( '' )  );
#39244=DIRECTION ( 'NONE',  ( 0.000000000000000000, -1.000000000000000000, 0.000000000000000000 ) ) ;
#39277=CIRCLE ( 'NONE', #37236, 6.349999999999999645 ) ;
#39280=DIRECTION ( 'NONE',  ( -1.000000000000000000, 0.000000000000000000, 0.000000000000000000 ) ) ;
#39284=CARTESIAN_POINT ( 'NONE',  ( -5.475330206976867231, 65.30181249999996851, 5.107412922131463695 ) ) ;
#39324=CARTESIAN_POINT ( 'NONE',  ( -12.21488373879589240, 55.24499999999999034, 5.016499999999999737 ) ) ;
#39328=LINE ( 'NONE', #28890, #14363 ) ;
#39335=CARTESIAN_POINT ( 'NONE',  ( -6.059261036834082681, 78.87450423423038615, -5.016499999999999737 ) ) ;
#39348=ADVANCED_FACE ( 'NONE', ( #25083 ), #41291, .T. ) ;
#39349=ORIENTED_EDGE ( 'NONE', *, *, #37275, .T. ) ;
#39352=FACE_OUTER_BOUND ( 'NONE', #12369, .T. ) ;
#39353=DIRECTION ( 'NONE',  ( 9.627370216492862708E-17, 1.000000000000000000, -0.000000000000000000 ) ) ;
#39362=ORIENTED_EDGE ( 'NONE', *, *, #644, .F. ) ;
#39365=ORIENTED_EDGE ( 'NONE', *, *, #35525, .T. ) ;
#39380=CARTESIAN_POINT ( 'NONE',  ( -5.570730988718118226, 56.51499999999999346, -4.419918923950581835 ) ) ;
#39388=CARTESIAN_POINT ( 'NONE',  ( -5.435468916197979006, 78.92497954178517716, -5.153742819109117690 ) ) ;
#39426=CARTESIAN_POINT ( 'NONE',  ( 17.14499999999999957, 71.11999999999999034, 5.016499999999999737 ) ) ;
#39427=CARTESIAN_POINT ( 'NONE',  ( -6.350000000000054712, 86.35999999999998522, 7.776507174585692163E-16 ) ) ;
#39428=CIRCLE ( 'NONE', #12902, 13.46199999999999442 ) ;
#39430=CARTESIAN_POINT ( 'NONE',  ( 10.28897677580358305, 56.51500000000000057, -4.381500000000000838 ) ) ;
#39433=EDGE_CURVE ( 'NONE', #19019, #27525, #14663, .T. ) ;
#39437=FACE_OUTER_BOUND ( 'NONE', #30796, .T. ) ;
#39444=DIRECTION ( 'NONE',  ( 0.7071067811865479058, -0.7071067811865472397, 0.000000000000000000 ) ) ;
#39448=DIRECTION ( 'NONE',  ( 9.627370216492862708E-17, 1.000000000000000000, -0.000000000000000000 ) ) ;
#39449=B_SPLINE_CURVE_WITH_KNOTS ( 'NONE', 3,
 ( #26561, #7820, #17177, #16964 ),
 .UNSPECIFIED., .F., .F.,
 ( 4, 4 ),
 ( 0.02839955696672240640, 1.000000000000000000 ),
 .UNSPECIFIED. ) ;
#39454=CARTESIAN_POINT ( 'NONE',  ( -16.42052266156670726, 59.67959903468464233, 5.072843609925764774 ) ) ;
#39456=CARTESIAN_POINT ( 'NONE',  ( -5.938360781727970661, 56.51499999999998636, 4.381499999999999950 ) ) ;
#39459=CARTESIAN_POINT ( 'NONE',  ( 6.059261036834405090, 56.51500000000000057, -4.381499999999999950 ) ) ;
#39468=DIRECTION ( 'NONE',  ( 1.000000000000000000, 0.000000000000000000, 0.000000000000000000 ) ) ;
#39470=CYLINDRICAL_SURFACE ( 'NONE', #20467, 6.349999999999999645 ) ;
#39498=CARTESIAN_POINT ( 'NONE',  ( -5.664977208693889210, 65.30181249999996851, 5.033228321271210781 ) ) ;
#39507=ORIENTED_EDGE ( 'NONE', *, *, #36141, .T. ) ;
#39518=B_SPLINE_CURVE_WITH_KNOTS ( 'NONE', 3,
 ( #7391, #4001, #33801, #36994, #36575, #16750, #27393, #14182, #7815, #4208 ),
 .UNSPECIFIED., .F., .F.,
 ( 4, 2, 2, 2, 4 ),
 ( 0.007397145391538723254, 0.008407694387831694122, 0.009418243384124664122, 0.01042879238041763412, 0.01143934137671060586 ),
 .UNSPECIFIED. ) ;
#39524=ORIENTED_EDGE ( 'NONE', *, *, #19746, .F. ) ;
#39535=ORIENTED_EDGE ( 'NONE', *, *, #38846, .F. ) ;
#39585=ORIENTED_EDGE ( 'NONE', *, *, #22386, .F. ) ;
#39587=CARTESIAN_POINT ( 'NONE',  ( -5.106395947886140263, 78.95054594174945350, 1.904999999999988258 ) ) ;
#39588=CARTESIAN_POINT ( 'NONE',  ( -10.32169608105474090, 17.14500000000000313, -4.040823496909975887 ) ) ;
#39603=DIRECTION ( 'NONE',  ( -1.000000000000000000, 0.000000000000000000, 0.000000000000000000 ) ) ;
#39604=VERTEX_POINT ( 'NONE', #15697 ) ;
#39616=CARTESIAN_POINT ( 'NONE',  ( -7.213960532367465817, 78.77618639008778700, -1.904999999999999583 ) ) ;
#39625=AXIS2_PLACEMENT_3D ( 'NONE', #2421, #25603, #5403 ) ;
#39639=VECTOR ( 'NONE', #2872, 1000.000000000000000 ) ;
#39641=FACE_OUTER_BOUND ( 'NONE', #26922, .T. ) ;
#39650=DIRECTION ( 'NONE',  ( 9.627370216492862708E-17, 1.000000000000000000, -0.000000000000000000 ) ) ;
#39678=EDGE_CURVE ( 'NONE', #12920, #26767, #20109, .T. ) ;
#39685=EDGE_CURVE ( 'NONE', #33497, #40327, #12931, .T. ) ;
#39695=EDGE_LOOP ( 'NONE', ( #8764, #34495, #15219, #5790 ) ) ;
#39713=CARTESIAN_POINT ( 'NONE',  ( -5.664977208693889210, 53.58606250000000415, 5.033228321271210781 ) ) ;
#39714=CARTESIAN_POINT ( 'NONE',  ( -5.322311913656985638, 57.15000000000021174, 5.239113282063311949 ) ) ;
#39733=DIRECTION ( 'NONE',  ( 0.8138664877804109299, 0.5810519254489895369, 0.000000000000000000 ) ) ;
#39749=ADVANCED_FACE ( 'NONE', ( #39352 ), #10372, .T. ) ;
#39763=CARTESIAN_POINT ( 'NONE',  ( -3.630816577625875226E-14, 57.14999999999999147, 0.000000000000000000 ) ) ;
#39777=CARTESIAN_POINT ( 'NONE',  ( 15.50061618130081165, 62.14374591690594940, -1.904999999999999583 ) ) ;
#39783=VERTEX_POINT ( 'NONE', #37001 ) ;
#39787=DIRECTION ( 'NONE',  ( 9.627370216492862708E-17, 1.000000000000000000, -0.000000000000000000 ) ) ;
#39789=EDGE_CURVE ( 'NONE', #25364, #20581, #14526, .T. ) ;
#39797=B_SPLINE_CURVE_WITH_KNOTS ( 'NONE', 3,
 ( #8584, #28174, #21547, #24541 ),
 .UNSPECIFIED., .F., .F.,
 ( 4, 4 ),
 ( 0.4905041263739763346, 1.000000000000000000 ),
 .UNSPECIFIED. ) ;
#39798=EDGE_CURVE ( 'NONE', #4652, #359, #39449, .T. ) ;
#39804=ORIENTED_EDGE ( 'NONE', *, *, #20228, .F. ) ;
#39821=ORIENTED_EDGE ( 'NONE', *, *, #12927, .F. ) ;
#39831=CARTESIAN_POINT ( 'NONE',  ( 14.79536922792820697, 61.64024183321802042, 1.904999999999990257 ) ) ;
#39847=AXIS2_PLACEMENT_3D ( 'NONE', #11724, #31529, #24712 ) ;
#39856=ORIENTED_EDGE ( 'NONE', *, *, #39433, .F. ) ;
#39864=CARTESIAN_POINT ( 'NONE',  ( 11.55299880265466506, 55.57741982016700177, 4.472382752598254463 ) ) ;
#39867=AXIS2_PLACEMENT_3D ( 'NONE', #40869, #31056, #28284 ) ;
#39872=CARTESIAN_POINT ( 'NONE',  ( -5.496588887047691330, 78.91991874857598077, 5.121802412194515597 ) ) ;
#39873=CARTESIAN_POINT ( 'NONE',  ( -10.62867326514809108, 56.48194529650092477, -4.405924061720180696 ) ) ;
#39882=LINE ( 'NONE', #32850, #34650 ) ;
#39885=CARTESIAN_POINT ( 'NONE',  ( -13.17422243436020857, 17.14499999999999957, -5.016499999999999737 ) ) ;
#39905=EDGE_LOOP ( 'NONE', ( #25473, #660, #11623, #9274 ) ) ;
#39906=VECTOR ( 'NONE', #20235, 1000.000000000000000 ) ;
#39912=EDGE_CURVE ( 'NONE', #27998, #42038, #14717, .T. ) ;
#39925=EDGE_CURVE ( 'NONE', #926, #25156, #23656, .T. ) ;
#39927=DIRECTION ( 'NONE',  ( -1.000000000000000000, 0.000000000000000000, 0.000000000000000000 ) ) ;
#39935=ORIENTED_EDGE ( 'NONE', *, *, #25682, .T. ) ;
#39947=ORIENTED_EDGE ( 'NONE', *, *, #23307, .F. ) ;
#39961=VERTEX_POINT ( 'NONE', #7609 ) ;
#39972=DIRECTION ( 'NONE',  ( -6.353134868986659519E-16, 1.000000000000000000, 0.000000000000000000 ) ) ;
#39978=CARTESIAN_POINT ( 'NONE',  ( 5.664977208693820820, 57.14999999999998437, 5.033228321271210781 ) ) ;
#39990=FACE_OUTER_BOUND ( 'NONE', #15711, .T. ) ;
#39992=B_SPLINE_CURVE_WITH_KNOTS ( 'NONE', 3,
 ( #22753, #19569, #3409, #16377, #29382, #222, #36628, #40042 ),
 .UNSPECIFIED., .F., .F.,
 ( 4, 2, 2, 4 ),
 ( 0.003986743484052247127, 0.004242962777773731133, 0.004499182071495215138, 0.005011620658938190087 ),
 .UNSPECIFIED. ) ;
#39999=ORIENTED_EDGE ( 'NONE', *, *, #30481, .F. ) ;
#40004=CARTESIAN_POINT ( 'NONE',  ( 5.860279866549846339, 57.15000000000084412, 5.019549989156823600 ) ) ;
#40017=CARTESIAN_POINT ( 'NONE',  ( -7.461250000000054783, 86.35999999999998522, 9.137395930138188390E-16 ) ) ;
#40023=CARTESIAN_POINT ( 'NONE',  ( -15.50061618130081165, 62.14374591690594940, -1.904999999999999583 ) ) ;
#40037=( GEOMETRIC_REPRESENTATION_CONTEXT ( 3 ) GLOBAL_UNCERTAINTY_ASSIGNED_CONTEXT ( ( #16317 ) ) GLOBAL_UNIT_ASSIGNED_CONTEXT ( ( #37942, #5793, #38372 ) ) REPRESENTATION_CONTEXT ( 'NONE', 'WORKASPACE' ) );
#40039=CARTESIAN_POINT ( 'NONE',  ( 5.348924234570989533, 56.51499999999999346, -4.492130288940734850 ) ) ;
#40042=CARTESIAN_POINT ( 'NONE',  ( -13.17422243436020857, 17.14499999999999957, -5.016499999999999737 ) ) ;
#40048=CARTESIAN_POINT ( 'NONE',  ( 5.965356522962838248, 77.01756249999996840, -5.016499999999999737 ) ) ;
#40076=FACE_OUTER_BOUND ( 'NONE', #21146, .T. ) ;
#40083=CARTESIAN_POINT ( 'NONE',  ( -5.385891243464945966, 78.92849802251097913, 5.190125708699868667 ) ) ;
#40105=AXIS2_PLACEMENT_3D ( 'NONE', #39454, #10256, #18839 ) ;
#40109=LINE ( 'NONE', #4540, #23365 ) ;
#40132=PLANE ( 'NONE',  #31444 ) ;
#40133=CARTESIAN_POINT ( 'NONE',  ( -11.66725022231030984, 17.14499999999999957, 5.016499999999999737 ) ) ;
#40139=LINE ( 'NONE', #11558, #16553 ) ;
#40143=CARTESIAN_POINT ( 'NONE',  ( 1.589478822742971486E-15, 16.51000000000000156, 0.000000000000000000 ) ) ;
#40144=ORIENTED_EDGE ( 'NONE', *, *, #21170, .F. ) ;
#40177=LINE ( 'NONE', #7796, #27015 ) ;
#40185=VECTOR ( 'NONE', #30929, 1000.000000000000000 ) ;
#40186=LINE ( 'NONE', #33789, #9958 ) ;
#40190=EDGE_LOOP ( 'NONE', ( #7774, #26409, #38505, #9094, #37663, #19002, #34599, #4276, #29725, #28659, #5297 ) ) ;
#40201=VECTOR ( 'NONE', #40791, 1000.000000000000000 ) ;
#40206=CARTESIAN_POINT ( 'NONE',  ( -13.85159022459153988, 12.96416000000000146, -5.016499999999999737 ) ) ;
#40221=CIRCLE ( 'NONE', #81, 14.09699999999999420 ) ;
#40232=CARTESIAN_POINT ( 'NONE',  ( 1.406077420118782567E-15, 14.60500000000000220, 0.000000000000000000 ) ) ;
#40261=CARTESIAN_POINT ( 'NONE',  ( 5.475330206976798841, 53.58606249999999704, -5.107412922131463695 ) ) ;
#40274=ORIENTED_EDGE ( 'NONE', *, *, #39912, .F. ) ;
#40277=EDGE_CURVE ( 'NONE', #8736, #37437, #13417, .T. ) ;
#40285=CARTESIAN_POINT ( 'NONE',  ( -5.965356522962929731, 57.14999999999999147, 5.016499999999999737 ) ) ;
#40299=CARTESIAN_POINT ( 'NONE',  ( -11.82906070755484507, 56.41571150956207958, -5.016499999999999737 ) ) ;
#40308=CARTESIAN_POINT ( 'NONE',  ( -5.817719362921545567, 56.51500000000001478, 4.384519708708647379 ) ) ;
#40317=CARTESIAN_POINT ( 'NONE',  ( -10.28897677580358305, 57.14999999999998437, -5.016499999999999737 ) ) ;
#40327=VERTEX_POINT ( 'NONE', #35477 ) ;
#40329=CARTESIAN_POINT ( 'NONE',  ( 1.222676017494593648E-15, 12.70000000000000284, 0.000000000000000000 ) ) ;
#40339=AXIS2_PLACEMENT_3D ( 'NONE', #829, #17616, #8045 ) ;
#40382=CARTESIAN_POINT ( 'NONE',  ( -4.997525182441658664, 56.61525291752814582, -5.184946129310926466 ) ) ;
#40390=CARTESIAN_POINT ( 'NONE',  ( 18.35410564743290607, 77.35382415001784295, 1.904999999999988480 ) ) ;
#40407=EDGE_LOOP ( 'NONE', ( #40677, #8877, #30531, #21647 ) ) ;
#40428=AXIS2_PLACEMENT_3D ( 'NONE', #17262, #20862, #21071 ) ;
#40433=CARTESIAN_POINT ( 'NONE',  ( -1.915954025944994433E-14, 30.83083951148100255, 1.904999999999999805 ) ) ;
#40434=CIRCLE ( 'NONE', #17273, 6.905625000000000568 ) ;
#40439=CYLINDRICAL_SURFACE ( 'NONE', #906, 7.461249999999999716 ) ;
#40441=CARTESIAN_POINT ( 'NONE',  ( 8.515285667870288113E-16, 8.844871939465425825, 0.000000000000000000 ) ) ;
#40442=CIRCLE ( 'NONE', #30204, 2.540000000000000480 ) ;
#40453=EDGE_CURVE ( 'NONE', #449, #18529, #9341, .T. ) ;
#40469=CARTESIAN_POINT ( 'NONE',  ( 6.059261036834384662, 88.73331249999999670, -5.016499999999999737 ) ) ;
#40486=EDGE_LOOP ( 'NONE', ( #6243, #41333, #37554, #27280 ) ) ;
#40491=EDGE_CURVE ( 'NONE', #37954, #1374, #35693, .T. ) ;
#40514=VECTOR ( 'NONE', #22547, 1000.000000000000000 ) ;
#40534=VERTEX_POINT ( 'NONE', #6502 ) ;
#40545=CARTESIAN_POINT ( 'NONE',  ( -11.48503488083560065, 55.92196062030127024, 5.016500000000108983 ) ) ;
#40548=CARTESIAN_POINT ( 'NONE',  ( -11.58677707360137532, 55.24499999999999034, 4.474811398758258285 ) ) ;
#40554=CARTESIAN_POINT ( 'NONE',  ( -5.224225543104921599, 57.14999999999898250, 5.327462464253450491 ) ) ;
#40571=CIRCLE ( 'NONE', #6563, 18.32410244842765934 ) ;
#40616=ORIENTED_EDGE ( 'NONE', *, *, #16981, .F. ) ;
#40632=ORIENTED_EDGE ( 'NONE', *, *, #30320, .T. ) ;
#40635=EDGE_CURVE ( 'NONE', #25156, #41231, #37738, .T. ) ;
#40646=EDGE_CURVE ( 'NONE', #25936, #35053, #41285, .T. ) ;
#40657=CARTESIAN_POINT ( 'NONE',  ( -12.69999999999999574, 17.14499999999999957, 0.000000000000000000 ) ) ;
#40659=ORIENTED_EDGE ( 'NONE', *, *, #4058, .F. ) ;
#40662=B_SPLINE_CURVE_WITH_KNOTS ( 'NONE', 3,
 ( #6928, #41879, #2899, #38464 ),
 .UNSPECIFIED., .F., .F.,
 ( 4, 4 ),
 ( 0.000000000000000000, 0.5094958736258470289 ),
 .UNSPECIFIED. ) ;
#40669=CARTESIAN_POINT ( 'NONE',  ( 5.965356522962860453, 53.58606249999999704, -5.016499999999999737 ) ) ;
#40677=ORIENTED_EDGE ( 'NONE', *, *, #4603, .F. ) ;
#40684=EDGE_LOOP ( 'NONE', ( #24698, #33167, #12225, #29696 ) ) ;
#40689=ORIENTED_EDGE ( 'NONE', *, *, #4501, .T. ) ;
#40691=CARTESIAN_POINT ( 'NONE',  ( 14.24929227862422465, 61.25037559889041461, -5.016500000000000625 ) ) ;
#40698=CARTESIAN_POINT ( 'NONE',  ( 10.45722248778855246, 56.52709681235302241, 5.016500000000865711 ) ) ;
#40701=ORIENTED_EDGE ( 'NONE', *, *, #19654, .F. ) ;
#40702=CARTESIAN_POINT ( 'NONE',  ( 19.68500000000000227, 71.11999999999999034, -1.904999999999999583 ) ) ;
#40706=CARTESIAN_POINT ( 'NONE',  ( -11.47253659098481293, 56.76836532675864788, -5.016499999999999737 ) ) ;
#40709=DIRECTION ( 'NONE',  ( 6.353134868986659519E-16, -1.000000000000000000, -0.000000000000000000 ) ) ;
#40728=EDGE_CURVE ( 'NONE', #21382, #37685, #16897, .T. ) ;
#40737=EDGE_CURVE ( 'NONE', #38115, #20977, #29411, .T. ) ;
#40739=VECTOR ( 'NONE', #3239, 1000.000000000000114 ) ;
#40740=CARTESIAN_POINT ( 'NONE',  ( -12.21488373879589240, 55.24499999999999034, 5.016499999999999737 ) ) ;
#40759=DIRECTION ( 'NONE',  ( 0.8138664877804109299, -0.5810519254489895369, 0.000000000000000000 ) ) ;
#40765=AXIS2_PLACEMENT_3D ( 'NONE', #37808, #15222, #17783 ) ;
#40766=EDGE_LOOP ( 'NONE', ( #14342, #15186, #28435, #11451 ) ) ;
#40778=CARTESIAN_POINT ( 'NONE',  ( 6.059261036834405978, 56.51500000000000057, 5.016500000000001513 ) ) ;
#40791=DIRECTION ( 'NONE',  ( -1.000000000000000000, -6.353134868986659519E-16, -0.000000000000000000 ) ) ;
#40808=PLANE ( 'NONE',  #40765 ) ;
#40821=CIRCLE ( 'NONE', #38743, 0.6350000000000001199 ) ;
#40823=CARTESIAN_POINT ( 'NONE',  ( -5.348924234571052594, 56.51499999999999346, -4.492130288940743732 ) ) ;
#40840=B_SPLINE_SURFACE_WITH_KNOTS ( 'NONE', 3, 1, ( 
 ( #36182, #7002 ),
 ( #3815, #16778 ),
 ( #29782, #13590 ),
 ( #26579, #39587 ) ),
 .UNSPECIFIED., .F., .F., .F.,
 ( 4, 4 ),
 ( 2, 2 ),
 ( 0.000000000000000000, 0.6118630412642116490 ),
 ( 0.000000000000000000, 1.000000000000000000 ),
 .UNSPECIFIED. ) ;
#40850=DIRECTION ( 'NONE',  ( -0.1469470846586743984, -9.335746474409589170E-17, -0.9891443546370349837 ) ) ;
#40855=DIRECTION ( 'NONE',  ( 0.1728608224830406603, -0.000000000000000000, -0.9849462604886047856 ) ) ;
#40863=DIRECTION ( 'NONE',  ( 1.000000000000000000, 0.000000000000000000, -1.224646799147351728E-16 ) ) ;
#40869=CARTESIAN_POINT ( 'NONE',  ( 12.21488373879589240, 71.11999999999999034, -4.381499999999999950 ) ) ;
#40888=VERTEX_POINT ( 'NONE', #35908 ) ;
#40900=VECTOR ( 'NONE', #10233, 1000.000000000000000 ) ;
#40903=DIRECTION ( 'NONE',  ( -6.146657985744592735E-16, 3.905054717696928257E-31, 1.000000000000000000 ) ) ;
#40905=ORIENTED_EDGE ( 'NONE', *, *, #39912, .T. ) ;
#40930=ORIENTED_EDGE ( 'NONE', *, *, #29088, .T. ) ;
#40931=CARTESIAN_POINT ( 'NONE',  ( 14.73199999999999754, 12.96302561210691628, 1.804149664503880250E-15 ) ) ;
#40933=SURFACE_STYLE_USAGE ( .BOTH. , #1962 ) ;
#40946=VECTOR ( 'NONE', #29004, 1000.000000000000000 ) ;
#40973=EDGE_CURVE ( 'NONE', #25156, #15597, #28605, .T. ) ;
#40984=ORIENTED_EDGE ( 'NONE', *, *, #25909, .F. ) ;
#40998=AXIS2_PLACEMENT_3D ( 'NONE', #3234, #16193, #41591 ) ;
#41004=DIRECTION ( 'NONE',  ( -9.627370216492862708E-17, -1.000000000000000000, 0.000000000000000000 ) ) ;
#41005=EDGE_CURVE ( 'NONE', #329, #18659, #35871, .T. ) ;
#41023=VECTOR ( 'NONE', #25907, 1000.000000000000000 ) ;
#41031=DIRECTION ( 'NONE',  ( 0.000000000000000000, 0.000000000000000000, 1.000000000000000000 ) ) ;
#41034=CARTESIAN_POINT ( 'NONE',  ( -7.461250000000053006, 83.56599999999998829, 9.137395930138198251E-16 ) ) ;
#41048=CARTESIAN_POINT ( 'NONE',  ( 4.792324638247207780, 56.51998046905276141, 4.972049999977001811 ) ) ;
#41051=CARTESIAN_POINT ( 'NONE',  ( 12.21488373879589240, 55.24500000000000455, -4.381499999999999950 ) ) ;
#41053=AXIS2_PLACEMENT_3D ( 'NONE', #8622, #31621, #5234 ) ;
#41059=CARTESIAN_POINT ( 'NONE',  ( 5.570375128628212380, 56.51500000000003610, -4.419987129958417249 ) ) ;
#41067=EDGE_CURVE ( 'NONE', #39604, #18019, #39797, .T. ) ;
#41091=VECTOR ( 'NONE', #34511, 1000.000000000000000 ) ;
#41099=ORIENTED_EDGE ( 'NONE', *, *, #10441, .F. ) ;
#41106=CARTESIAN_POINT ( 'NONE',  ( -5.475330206976867231, 57.14999999999999147, 5.107412922131463695 ) ) ;
#41117=ORIENTED_EDGE ( 'NONE', *, *, #26125, .T. ) ;
#41126=DIRECTION ( 'NONE',  ( 1.000000000000000000, 0.000000000000000000, 0.000000000000000000 ) ) ;
#41157=LINE ( 'NONE', #24159, #36710 ) ;
#41193=EDGE_CURVE ( 'NONE', #35053, #15866, #28062, .T. ) ;
#41210=ADVANCED_FACE ( 'NONE', ( #37975 ), #8800, .F. ) ;
#41215=EDGE_CURVE ( 'NONE', #21005, #24253, #41312, .T. ) ;
#41218=CARTESIAN_POINT ( 'NONE',  ( 17.14500000000001023, 57.15000000000000568, -5.016499999999999737 ) ) ;
#41227=ORIENTED_EDGE ( 'NONE', *, *, #34053, .T. ) ;
#41231=VERTEX_POINT ( 'NONE', #31583 ) ;
#41243=CARTESIAN_POINT ( 'NONE',  ( -6.059261036834474368, 56.51499999999998636, -4.381499999999999950 ) ) ;
#41258=VECTOR ( 'NONE', #30850, 1000.000000000000114 ) ;
#41263=AXIS2_PLACEMENT_3D ( 'NONE', #27068, #39650, #26857 ) ;
#41268=EDGE_CURVE ( 'NONE', #27998, #18952, #19113, .T. ) ;
#41273=CARTESIAN_POINT ( 'NONE',  ( 6.059261036834405978, 57.14999999999999858, -5.016499999999999737 ) ) ;
#41285=B_SPLINE_CURVE_WITH_KNOTS ( 'NONE', 5,
 ( #552, #3538, #10325, #29710, #26728, #19902, #16705, #17129 ),
 .UNSPECIFIED., .F., .F.,
 ( 6, 2, 6 ),
 ( 0.000000000000000000, 0.0004921095964230317449, 0.0009842191928460634898 ),
 .UNSPECIFIED. ) ;
#41287=CARTESIAN_POINT ( 'NONE',  ( 6.113380087472956159E-17, 0.6350000000000001199, 0.000000000000000000 ) ) ;
#41291=CYLINDRICAL_SURFACE ( 'NONE', #39867, 0.6350000000000001199 ) ;
#41294=DIRECTION ( 'NONE',  ( -1.000000000000000000, -6.353134868986659519E-16, 6.146657985744592735E-16 ) ) ;
#41305=ORIENTED_EDGE ( 'NONE', *, *, #16531, .T. ) ;
#41312=CIRCLE ( 'NONE', #15443, 6.350000000000004974 ) ;
#41313=ORIENTED_EDGE ( 'NONE', *, *, #363, .T. ) ;
#41320=CARTESIAN_POINT ( 'NONE',  ( 5.579075174912572876, 56.51499999999997925, 4.418274828058815551 ) ) ;
#41325=CARTESIAN_POINT ( 'NONE',  ( 6.059261036834400649, 64.39150124418100063, -5.016499999999999737 ) ) ;
#41326=CARTESIAN_POINT ( 'NONE',  ( -11.32678463655001266, 56.02547433970818958, 4.456118031212522368 ) ) ;
#41330=DIRECTION ( 'NONE',  ( -1.000000000000000000, 0.000000000000000000, 0.000000000000000000 ) ) ;
#41333=ORIENTED_EDGE ( 'NONE', *, *, #40646, .T. ) ;
#41348=PLANE ( 'NONE',  #3365 ) ;
#41358=ORIENTED_EDGE ( 'NONE', *, *, #23354, .F. ) ;
#41359=ORIENTED_EDGE ( 'NONE', *, *, #13430, .T. ) ;
#41374=( BOUNDED_SURFACE ( )  B_SPLINE_SURFACE ( 3, 2, ( 
 ( #18086, #1930, #18711 ),
 ( #5543, #27892, #8936 ),
 ( #31721, #37698, #8520 ),
 ( #32554, #29361, #13384 ),
 ( #22730, #23152, #199 ),
 ( #22524, #2972, #16139 ),
 ( #26372, #16786, #36189 ),
 ( #35761, #6788, #6576 ),
 ( #39380, #19544, #19977 ),
 ( #415, #10183, #38955 ),
 ( #29581, #19754, #9765 ),
 ( #32346, #9970, #627 ) ),
 .UNSPECIFIED., .F., .F., .T. ) 
 B_SPLINE_SURFACE_WITH_KNOTS ( ( 4, 2, 2, 2, 2, 4 ),
 ( 3, 3 ),
 ( -1.344410693882025498E-17, 0.0001838632285168812104, 0.0003677264570337758650, 0.0007354529140675651741, 0.001103179371101354429, 0.001470905828135143792 ),
 ( 0.000000000000000000, 1.000000000000000000 ),
 .UNSPECIFIED. ) 
 GEOMETRIC_REPRESENTATION_ITEM ( )  RATIONAL_B_SPLINE_SURFACE ( (
 ( 1.000000000000000000, 0.7071067811865514585, 1.000000000000000000),
 ( 1.000000000000000000, 0.7071067811865514585, 1.000000000000000000),
 ( 1.000000000000000000, 0.7071067811865436870, 1.000000000000000000),
 ( 1.000000000000000000, 0.7071067811865436870, 1.000000000000000000),
 ( 1.000000000000000000, 0.7071067811865436870, 1.000000000000000000),
 ( 1.000000000000000000, 0.7071067811865436870, 1.000000000000000000),
 ( 1.000000000000000000, 0.7071067811865514585, 1.000000000000000000),
 ( 1.000000000000000000, 0.7071067811865514585, 1.000000000000000000),
 ( 1.000000000000000000, 0.7071067811865514585, 1.000000000000000000),
 ( 1.000000000000000000, 0.7071067811865514585, 1.000000000000000000),
 ( 1.000000000000000000, 0.7071067811865514585, 1.000000000000000000),
 ( 1.000000000000000000, 0.7071067811865514585, 1.000000000000000000) ) ) 
 REPRESENTATION_ITEM ( '' )  SURFACE ( )  );
#41379=DIRECTION ( 'NONE',  ( -1.000000000000000000, 0.000000000000000000, 0.000000000000000000 ) ) ;
#41408=ORIENTED_EDGE ( 'NONE', *, *, #31595, .T. ) ;
#41421=EDGE_CURVE ( 'NONE', #1422, #359, #36238, .T. ) ;
#41422=ADVANCED_FACE ( 'NONE', ( #183 ), #31894, .T. ) ;
#41441=ORIENTED_EDGE ( 'NONE', *, *, #34197, .T. ) ;
#41457=DIRECTION ( 'NONE',  ( -1.000000000000000000, -9.299908063537918137E-16, 0.000000000000000000 ) ) ;
#41459=ORIENTED_EDGE ( 'NONE', *, *, #18079, .T. ) ;
#41473=PLANE ( 'NONE',  #7060 ) ;
#41485=CARTESIAN_POINT ( 'NONE',  ( 5.638141748396324537, 57.14999999999959357, -5.060111600445807767 ) ) ;
#41504=CARTESIAN_POINT ( 'NONE',  ( 6.604684614740960136, 78.82897922428260529, -3.487443616724450468 ) ) ;
#41510=CARTESIAN_POINT ( 'NONE',  ( 5.115874721082195542, 56.51499999999995083, 4.603382018213770799 ) ) ;
#41523=B_SPLINE_CURVE_WITH_KNOTS ( 'NONE', 3,
 ( #20247, #23655, #1109, #14077, #23871, #20671 ),
 .UNSPECIFIED., .F., .F.,
 ( 4, 2, 4 ),
 ( -7.295512719012818938E-06, 0.0003601880853723633683, 0.0007276716834637395352 ),
 .UNSPECIFIED. ) ;
#41535=CARTESIAN_POINT ( 'NONE',  ( -11.47253659098475254, 56.76836532675849156, 5.016499999999999737 ) ) ;
#41579=CIRCLE ( 'NONE', #8235, 6.985000000000000320 ) ;
#41591=DIRECTION ( 'NONE',  ( 0.000000000000000000, 0.000000000000000000, 1.000000000000000000 ) ) ;
#41603=DIRECTION ( 'NONE',  ( -1.000000000000000000, 1.177520686924251719E-16, 0.000000000000000000 ) ) ;
#41633=AXIS2_PLACEMENT_3D ( 'NONE', #41287, #27857, #34678 ) ;
#41636=B_SPLINE_CURVE_WITH_KNOTS ( 'NONE', 3,
 ( #35518, #19310, #32314, #9319, #28697, #16107 ),
 .UNSPECIFIED., .F., .F.,
 ( 4, 2, 4 ),
 ( 0.000000000000000000, 0.5000000000000000000, 1.000000000000000000 ),
 .UNSPECIFIED. ) ;
#41640=CARTESIAN_POINT ( 'NONE',  ( 6.349999999999945466, 85.80437499999999318, 0.000000000000000000 ) ) ;
#41650=CARTESIAN_POINT ( 'NONE',  ( -5.475330206976889436, 88.73331249999999670, -5.107412922131463695 ) ) ;
#41662=CARTESIAN_POINT ( 'NONE',  ( 9.638062024671789629, 56.51500000000000057, 4.786355703798467734E-15 ) ) ;
#41666=CARTESIAN_POINT ( 'NONE',  ( 7.213960532363564937, 86.35999999999998522, -1.904999999999999805 ) ) ;
#41671=ORIENTED_EDGE ( 'NONE', *, *, #17540, .T. ) ;
#41689=VECTOR ( 'NONE', #17331, 1000.000000000000000 ) ;
#41708=ORIENTED_EDGE ( 'NONE', *, *, #37275, .F. ) ;
#41711=DIRECTION ( 'NONE',  ( 1.000000000000000000, 0.000000000000000000, 0.000000000000000000 ) ) ;
#41713=CARTESIAN_POINT ( 'NONE',  ( -14.79536922792821052, 61.64024183321802752, 1.905000000000008686 ) ) ;
#41730=CIRCLE ( 'NONE', #15194, 7.461249999999999716 ) ;
#41733=EDGE_LOOP ( 'NONE', ( #20956, #29243, #19094, #12092 ) ) ;
#41737=CARTESIAN_POINT ( 'NONE',  ( -10.92199999999999704, 16.51000000000000156, 5.016499999999999737 ) ) ;
#41746=CARTESIAN_POINT ( 'NONE',  ( -10.45722248778793428, 56.52709681235294426, 5.016499999999999737 ) ) ;
#41751=VECTOR ( 'NONE', #21416, 1000.000000000000114 ) ;
#41763=CYLINDRICAL_SURFACE ( 'NONE', #29894, 0.6349999999999966782 ) ;
#41795=VERTEX_POINT ( 'NONE', #37993 ) ;
#41798=FACE_OUTER_BOUND ( 'NONE', #13487, .T. ) ;
#41826=ORIENTED_EDGE ( 'NONE', *, *, #1086, .F. ) ;
#41827=CARTESIAN_POINT ( 'NONE',  ( 5.475330206976798841, 65.30181249999998272, 5.107412922131463695 ) ) ;
#41835=EDGE_LOOP ( 'NONE', ( #17784, #40930, #28365, #3228 ) ) ;
#41840=DIRECTION ( 'NONE',  ( 1.000000000000000000, 0.000000000000000000, 0.000000000000000000 ) ) ;
#41864=CARTESIAN_POINT ( 'NONE',  ( -5.305748947172302721, 77.01756249999996840, -5.247078976224250013 ) ) ;
#41876=CARTESIAN_POINT ( 'NONE',  ( 5.249547376965405299, 56.51500000000000767, -4.563748390642682118 ) ) ;
#41879=CARTESIAN_POINT ( 'NONE',  ( 15.15189561879875768, 77.97492127061545375, 1.904999999999999583 ) ) ;
#41882=CARTESIAN_POINT ( 'NONE',  ( 10.28897677580358128, 57.14999999999999858, 4.381499999999999950 ) ) ;
#41883=LINE ( 'NONE', #3110, #24092 ) ;
#41910=DIRECTION ( 'NONE',  ( 1.000000000000000000, 0.000000000000000000, 0.000000000000000000 ) ) ;
#41933=AXIS2_PLACEMENT_3D ( 'NONE', #28746, #9365, #28541 ) ;
#41935=VECTOR ( 'NONE', #12450, 1000.000000000000000 ) ;
#41937=VECTOR ( 'NONE', #33683, 1000.000000000000000 ) ;
#41944=DIRECTION ( 'NONE',  ( 0.000000000000000000, -1.000000000000000000, 0.000000000000000000 ) ) ;
#41947=EDGE_CURVE ( 'NONE', #29906, #37417, #15816, .T. ) ;
#41959=ORIENTED_EDGE ( 'NONE', *, *, #26593, .F. ) ;
#41968=CARTESIAN_POINT ( 'NONE',  ( 14.39766717389552042, 60.87500489999898434, -1.904999999999999583 ) ) ;
#41971=DIRECTION ( 'NONE',  ( 0.1469470846586743984, 9.335746474409589170E-17, -0.9891443546370349837 ) ) ;
#41989=( BOUNDED_CURVE ( )  B_SPLINE_CURVE ( 3, ( #41662, #28651, #19474, #29496 ),
 .UNSPECIFIED., .F., .T. ) 
 B_SPLINE_CURVE_WITH_KNOTS ( ( 4, 4 ),
 ( 1.570796326794895892, 3.141592653589793560 ),
 .UNSPECIFIED. ) 
 CURVE ( )  GEOMETRIC_REPRESENTATION_ITEM ( )  RATIONAL_B_SPLINE_CURVE ( ( 1.000000000000000000, 0.8047378541243646044, 0.8047378541243646044, 1.000000000000000000 ) ) 
 REPRESENTATION_ITEM ( '' )  );
#42011=ADVANCED_FACE ( 'NONE', ( #8392 ), #21354, .F. ) ;
#42021=CARTESIAN_POINT ( 'NONE',  ( 13.85159022459153988, 12.96416000000000146, 5.016499999999999737 ) ) ;
#42026=TOROIDAL_SURFACE ( 'NONE', #41933, 6.905624999999998792, 0.5556250000000014788 ) ;
#42029=CARTESIAN_POINT ( 'NONE',  ( 5.965356522962838248, 88.73331249999999670, 5.016499999999999737 ) ) ;
#42031=ORIENTED_EDGE ( 'NONE', *, *, #18745, .F. ) ;
#42038=VERTEX_POINT ( 'NONE', #18800 ) ;
#42048=AXIS2_PLACEMENT_3D ( 'NONE', #22403, #13262, #3269 ) ;
#42050=ORIENTED_EDGE ( 'NONE', *, *, #36776, .F. ) ;
#42064=FACE_OUTER_BOUND ( 'NONE', #20067, .T. ) ;
#42072=DIRECTION ( 'NONE',  ( 9.627370216492862708E-17, 1.000000000000000000, -0.000000000000000000 ) ) ;
#42078=ORIENTED_EDGE ( 'NONE', *, *, #40453, .F. ) ;
#42093=FACE_OUTER_BOUND ( 'NONE', #18273, .T. ) ;
#42104=EDGE_CURVE ( 'NONE', #27131, #31875, #18192, .T. ) ;
#42109=FACE_OUTER_BOUND ( 'NONE', #13924, .T. ) ;
#42116=DIRECTION ( 'NONE',  ( -1.000000000000000000, 0.000000000000000000, -5.975917486140574681E-16 ) ) ;
#42131=VERTEX_POINT ( 'NONE', #16228 ) ;
#42135=CARTESIAN_POINT ( 'NONE',  ( -11.58677707360137532, 17.14500000000000313, -4.474811398758258285 ) ) ;
#42142=AXIS2_PLACEMENT_3D ( 'NONE', #1533, #14076, #16854 ) ;
#42143=CARTESIAN_POINT ( 'NONE',  ( 5.177913976931212581, 57.14999999999999147, 5.372099999999999653 ) ) ;
#42153=DIRECTION ( 'NONE',  ( 9.627370216492862708E-17, 1.000000000000000000, -0.000000000000000000 ) ) ;
ENDSEC;
END-ISO-10303-21;
